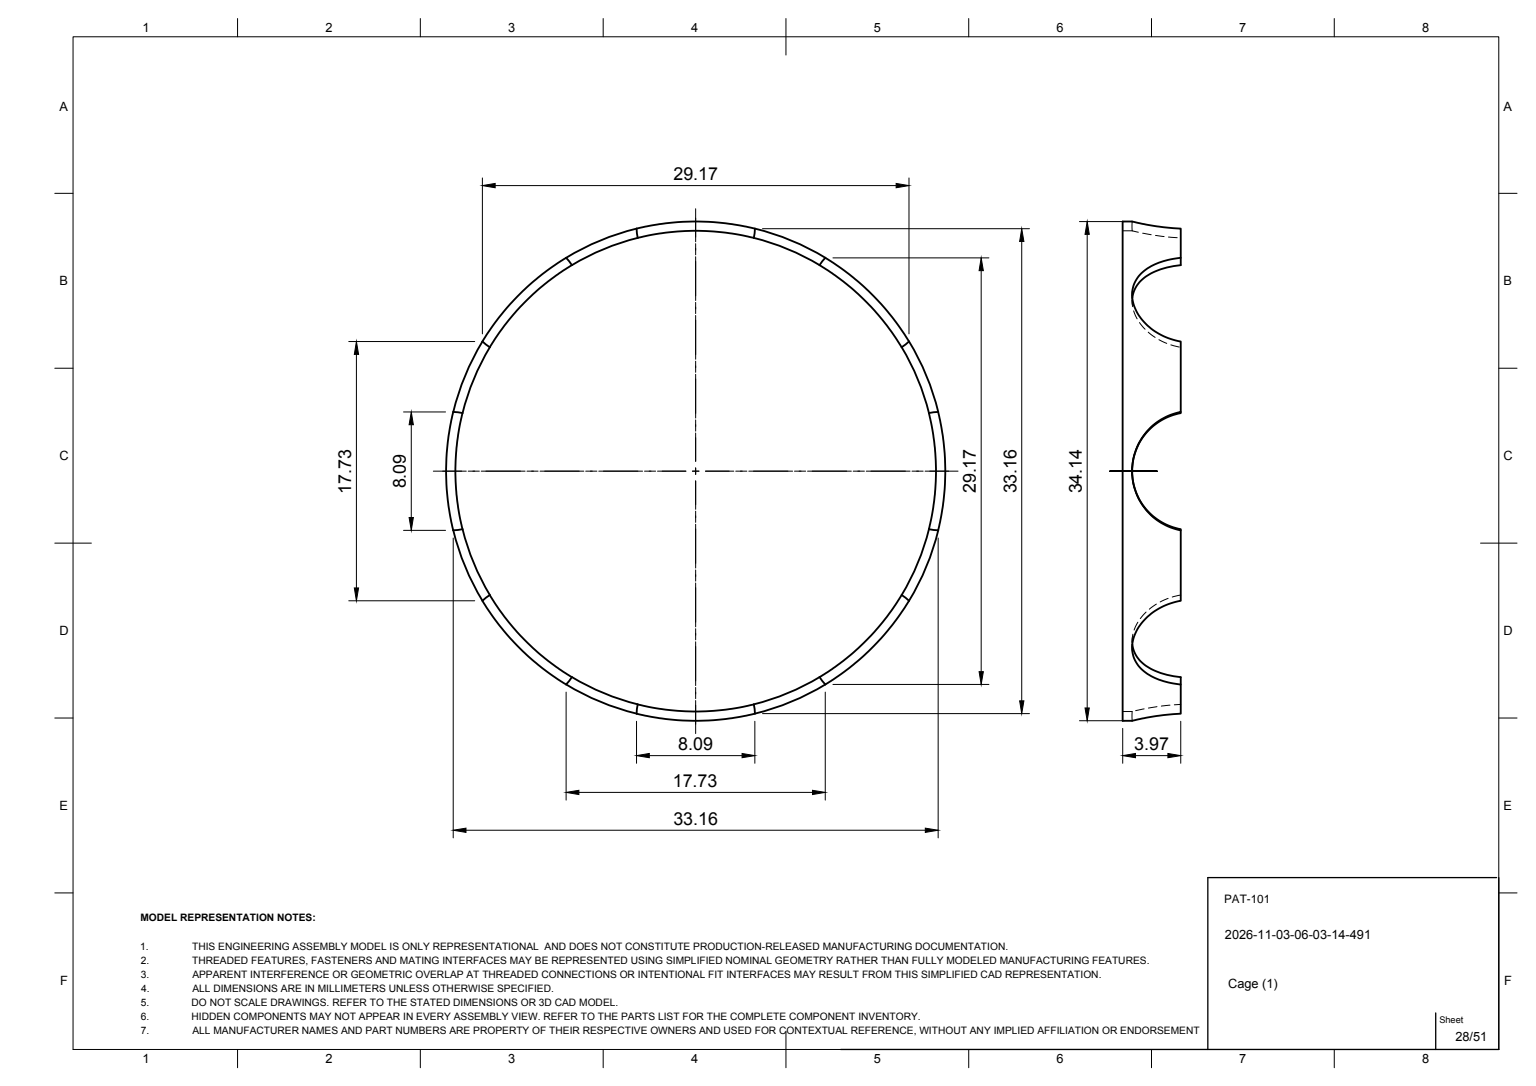
ISO-10303-21;
HEADER;
/* Generated by software containing ST-Developer
 * from STEP Tools, Inc. (www.steptools.com) 
 */

FILE_DESCRIPTION(
/* description */ ('Spur gear reduction stage 2-1 on bearing plates'),
/* implementation_level */ '2;1');

FILE_NAME(
/* name */ 'Cage (1).step',
/* time_stamp */ '2026-10-28T03:22:07-07:00',
/* author */ (''),
/* organization */ (''),
/* preprocessor_version */ 'ST-DEVELOPER v20.2',
/* originating_system */ 'Autodesk Translation Framework v15.17.0.0',
/* authorisation */ '');

FILE_SCHEMA (('AUTOMOTIVE_DESIGN { 1 0 10303 214 3 1 1 }'));
ENDSEC;

DATA;
#10=MECHANICAL_DESIGN_GEOMETRIC_PRESENTATION_REPRESENTATION('',(#982),#53909);
#681=B_SPLINE_CURVE_WITH_KNOTS('',3,(#17332,#17333,#17334,#17335,#17336,
#17337,#17338,#17339,#17340,#17341,#17342,#17343,#17344,#17345,#17346,#17347,
#17348,#17349,#17350,#17351,#17352,#17353),.UNSPECIFIED.,.F.,.F.,(4,2,2,
2,2,2,2,2,2,2,4),(0.0789094028588958,0.210573405340968,0.315860108011452,
0.421146810681936,0.522142632548711,0.623138454415485,0.72413427628226,
0.825130098149035,0.930416800819519,1.03570350349,1.16736750597208),
 .UNSPECIFIED.);
#682=B_SPLINE_CURVE_WITH_KNOTS('',3,(#17357,#17358,#17359,#17360,#17361,
#17362,#17363,#17364,#17365,#17366,#17367,#17368,#17369,#17370,#17371,#17372,
#17373,#17374,#17375,#17376,#17377,#17378),.UNSPECIFIED.,.F.,.F.,(4,2,2,
2,2,2,2,2,2,2,4),(0.0774793363974613,0.142088896491891,0.284177792983782,
0.411119756996526,0.514392970548519,0.617666184100513,0.720939397652506,
0.8242126112045,0.951154575217244,1.09324347170913,1.15785303180356),
 .UNSPECIFIED.);
#683=B_SPLINE_CURVE_WITH_KNOTS('',3,(#17384,#17385,#17386,#17387,#17388,
#17389,#17390,#17391,#17392,#17393,#17394,#17395,#17396,#17397,#17398,#17399,
#17400,#17401,#17402,#17403,#17404,#17405),.UNSPECIFIED.,.F.,.F.,(4,2,2,
2,2,2,2,2,2,2,4),(0.0774793363974613,0.142088896491891,0.284177792983782,
0.411119756996525,0.514392970548519,0.617666184100513,0.720939397652506,
0.8242126112045,0.951154575217243,1.09324347170913,1.15785303180356),
 .UNSPECIFIED.);
#684=B_SPLINE_CURVE_WITH_KNOTS('',3,(#17409,#17410,#17411,#17412,#17413,
#17414,#17415,#17416,#17417,#17418,#17419,#17420,#17421,#17422,#17423,#17424,
#17425,#17426,#17427,#17428,#17429,#17430),.UNSPECIFIED.,.F.,.F.,(4,2,2,
2,2,2,2,2,2,2,4),(0.0774793363974614,0.142088896491891,0.284177792983781,
0.411119756996525,0.514392970548519,0.617666184100512,0.720939397652506,
0.824212611204499,0.951154575217243,1.09324347170913,1.15785303180356),
 .UNSPECIFIED.);
#685=B_SPLINE_CURVE_WITH_KNOTS('',3,(#17434,#17435,#17436,#17437,#17438,
#17439,#17440,#17441,#17442,#17443,#17444,#17445),.UNSPECIFIED.,.F.,.F.,
(4,2,2,2,2,4),(0.0774793363974613,0.142088896491891,0.284177792983781,0.411119756996525,
0.514392970548519,0.617666184100512),.UNSPECIFIED.);
#686=B_SPLINE_CURVE_WITH_KNOTS('',3,(#17450,#17451,#17452,#17453,#17454,
#17455,#17456,#17457,#17458,#17459,#17460,#17461),.UNSPECIFIED.,.F.,.F.,
(4,2,2,2,2,4),(0.617666184100512,0.720939397652506,0.824212611204499,0.951154575217243,
1.09324347170913,1.15785303180356),.UNSPECIFIED.);
#687=B_SPLINE_CURVE_WITH_KNOTS('',3,(#17465,#17466,#17467,#17468,#17469,
#17470,#17471,#17472,#17473,#17474,#17475,#17476,#17477,#17478,#17479,#17480,
#17481,#17482,#17483,#17484,#17485,#17486),.UNSPECIFIED.,.F.,.F.,(4,2,2,
2,2,2,2,2,2,2,4),(0.0774793363974613,0.142088896491891,0.284177792983782,
0.411119756996526,0.514392970548519,0.617666184100513,0.720939397652507,
0.8242126112045,0.951154575217245,1.09324347170914,1.15785303180356),
 .UNSPECIFIED.);
#688=B_SPLINE_CURVE_WITH_KNOTS('',3,(#17490,#17491,#17492,#17493,#17494,
#17495,#17496,#17497,#17498,#17499,#17500,#17501,#17502,#17503,#17504,#17505,
#17506,#17507,#17508,#17509,#17510,#17511),.UNSPECIFIED.,.F.,.F.,(4,2,2,
2,2,2,2,2,2,2,4),(0.0774793363974613,0.142088896491891,0.284177792983782,
0.411119756996526,0.514392970548519,0.617666184100513,0.720939397652506,
0.824212611204499,0.951154575217243,1.09324347170913,1.15785303180356),
 .UNSPECIFIED.);
#689=B_SPLINE_CURVE_WITH_KNOTS('',3,(#17515,#17516,#17517,#17518,#17519,
#17520,#17521,#17522,#17523,#17524,#17525,#17526,#17527,#17528,#17529,#17530,
#17531,#17532,#17533,#17534,#17535,#17536),.UNSPECIFIED.,.F.,.F.,(4,2,2,
2,2,2,2,2,2,2,4),(0.0774793363974613,0.142088896491891,0.284177792983782,
0.411119756996526,0.514392970548519,0.617666184100513,0.720939397652506,
0.8242126112045,0.951154575217244,1.09324347170913,1.15785303180356),
 .UNSPECIFIED.);
#690=B_SPLINE_CURVE_WITH_KNOTS('',3,(#17540,#17541,#17542,#17543,#17544,
#17545,#17546,#17547,#17548,#17549,#17550,#17551,#17552,#17553,#17554,#17555,
#17556,#17557,#17558,#17559,#17560,#17561),.UNSPECIFIED.,.F.,.F.,(4,2,2,
2,2,2,2,2,2,2,4),(0.0774793363974613,0.142088896491891,0.284177792983782,
0.411119756996526,0.514392970548519,0.617666184100513,0.720939397652506,
0.8242126112045,0.951154575217243,1.09324347170913,1.15785303180356),
 .UNSPECIFIED.);
#691=B_SPLINE_CURVE_WITH_KNOTS('',3,(#17569,#17570,#17571,#17572,#17573,
#17574,#17575,#17576,#17577,#17578,#17579,#17580,#17581,#17582,#17583,#17584,
#17585,#17586,#17587,#17588,#17589,#17590),.UNSPECIFIED.,.F.,.F.,(4,2,2,
2,2,2,2,2,2,2,4),(0.0789094028588958,0.210573405340968,0.315860108011452,
0.421146810681936,0.522142632548711,0.623138454415485,0.72413427628226,
0.825130098149035,0.930416800819519,1.03570350349,1.16736750597208),
 .UNSPECIFIED.);
#692=B_SPLINE_CURVE_WITH_KNOTS('',3,(#17598,#17599,#17600,#17601,#17602,
#17603,#17604,#17605,#17606,#17607,#17608,#17609,#17610,#17611,#17612,#17613,
#17614,#17615,#17616,#17617,#17618,#17619),.UNSPECIFIED.,.F.,.F.,(4,2,2,
2,2,2,2,2,2,2,4),(0.0789094028588958,0.210573405340969,0.315860108011453,
0.421146810681937,0.522142632548712,0.623138454415486,0.724134276282261,
0.825130098149035,0.930416800819519,1.03570350349,1.16736750597208),
 .UNSPECIFIED.);
#693=B_SPLINE_CURVE_WITH_KNOTS('',3,(#17628,#17629,#17630,#17631,#17632,
#17633,#17634,#17635,#17636,#17637,#17638,#17639),.UNSPECIFIED.,.F.,.F.,
(4,2,2,2,2,4),(0.0789094028588958,0.210573405340968,0.315860108011452,0.421146810681937,
0.522142632548711,0.623138454415486),.UNSPECIFIED.);
#694=B_SPLINE_CURVE_WITH_KNOTS('',3,(#17641,#17642,#17643,#17644,#17645,
#17646,#17647,#17648,#17649,#17650,#17651,#17652),.UNSPECIFIED.,.F.,.F.,
(4,2,2,2,2,4),(0.623138454415486,0.72413427628226,0.825130098149035,0.930416800819519,
1.03570350349,1.16736750597208),.UNSPECIFIED.);
#695=B_SPLINE_CURVE_WITH_KNOTS('',3,(#17659,#17660,#17661,#17662,#17663,
#17664,#17665,#17666,#17667,#17668,#17669,#17670,#17671,#17672,#17673,#17674,
#17675,#17676,#17677,#17678,#17679,#17680),.UNSPECIFIED.,.F.,.F.,(4,2,2,
2,2,2,2,2,2,2,4),(0.0789094028588958,0.210573405340968,0.315860108011452,
0.421146810681936,0.522142632548711,0.623138454415486,0.72413427628226,
0.825130098149035,0.930416800819519,1.03570350349,1.16736750597208),
 .UNSPECIFIED.);
#696=B_SPLINE_CURVE_WITH_KNOTS('',3,(#17688,#17689,#17690,#17691,#17692,
#17693,#17694,#17695,#17696,#17697,#17698,#17699,#17700,#17701,#17702,#17703,
#17704,#17705,#17706,#17707,#17708,#17709),.UNSPECIFIED.,.F.,.F.,(4,2,2,
2,2,2,2,2,2,2,4),(0.0789094028588957,0.210573405340968,0.315860108011452,
0.421146810681936,0.522142632548711,0.623138454415485,0.72413427628226,
0.825130098149035,0.930416800819519,1.03570350349,1.16736750597207),
 .UNSPECIFIED.);
#697=B_SPLINE_CURVE_WITH_KNOTS('',3,(#17717,#17718,#17719,#17720,#17721,
#17722,#17723,#17724,#17725,#17726,#17727,#17728,#17729,#17730,#17731,#17732,
#17733,#17734,#17735,#17736,#17737,#17738),.UNSPECIFIED.,.F.,.F.,(4,2,2,
2,2,2,2,2,2,2,4),(0.0789094028588958,0.210573405340968,0.315860108011452,
0.421146810681936,0.522142632548711,0.623138454415486,0.72413427628226,
0.825130098149035,0.930416800819519,1.03570350349,1.16736750597208),
 .UNSPECIFIED.);
#698=B_SPLINE_CURVE_WITH_KNOTS('',3,(#17747,#17748,#17749,#17750,#17751,
#17752,#17753,#17754,#17755,#17756,#17757,#17758,#17759,#17760,#17761,#17762,
#17763,#17764,#17765,#17766,#17767,#17768),.UNSPECIFIED.,.F.,.F.,(4,2,2,
2,2,2,2,2,2,2,4),(0.0789094028588958,0.210573405340968,0.315860108011452,
0.421146810681936,0.522142632548711,0.623138454415485,0.72413427628226,
0.825130098149035,0.930416800819519,1.03570350349,1.16736750597208),
 .UNSPECIFIED.);
#817=SPHERICAL_SURFACE('',#12340,0.412776);
#818=SPHERICAL_SURFACE('',#12356,0.412776);
#819=SPHERICAL_SURFACE('',#12361,0.412776);
#820=SPHERICAL_SURFACE('',#12366,0.412776);
#821=SPHERICAL_SURFACE('',#12371,0.412776);
#822=SPHERICAL_SURFACE('',#12376,0.412776);
#823=SPHERICAL_SURFACE('',#12381,0.412776);
#824=SPHERICAL_SURFACE('',#12389,0.412776);
#882=SHAPE_REPRESENTATION_RELATIONSHIP('SRR','None',#54111,#925);
#925=ADVANCED_BREP_SHAPE_REPRESENTATION('',(#1038),#53885);
#982=STYLED_ITEM('',(#54397),#1038);
#1038=MANIFOLD_SOLID_BREP('Continuous crown cage',#11308);
#1191=FACE_BOUND('',#2536,.T.);
#1334=PLANE('',#12353);
#1335=PLANE('',#12358);
#1336=PLANE('',#12363);
#1337=PLANE('',#12368);
#1338=PLANE('',#12373);
#1339=PLANE('',#12378);
#1340=PLANE('',#12387);
#1341=PLANE('',#12391);
#1342=PLANE('',#12392);
#1739=FACE_OUTER_BOUND('',#2518,.T.);
#1740=FACE_OUTER_BOUND('',#2519,.T.);
#1741=FACE_OUTER_BOUND('',#2520,.T.);
#1742=FACE_OUTER_BOUND('',#2521,.T.);
#1743=FACE_OUTER_BOUND('',#2522,.T.);
#1744=FACE_OUTER_BOUND('',#2523,.T.);
#1745=FACE_OUTER_BOUND('',#2524,.T.);
#1746=FACE_OUTER_BOUND('',#2525,.T.);
#1747=FACE_OUTER_BOUND('',#2526,.T.);
#1748=FACE_OUTER_BOUND('',#2527,.T.);
#1749=FACE_OUTER_BOUND('',#2528,.T.);
#1750=FACE_OUTER_BOUND('',#2529,.T.);
#1751=FACE_OUTER_BOUND('',#2530,.T.);
#1752=FACE_OUTER_BOUND('',#2531,.T.);
#1753=FACE_OUTER_BOUND('',#2532,.T.);
#1754=FACE_OUTER_BOUND('',#2533,.T.);
#1755=FACE_OUTER_BOUND('',#2534,.T.);
#1756=FACE_OUTER_BOUND('',#2535,.T.);
#1757=FACE_OUTER_BOUND('',#2537,.T.);
#2518=EDGE_LOOP('',(#8286,#8287,#8288,#8289));
#2519=EDGE_LOOP('',(#8290,#8291,#8292,#8293,#8294,#8295,#8296,#8297,#8298,
#8299,#8300,#8301,#8302,#8303,#8304,#8305,#8306,#8307,#8308,#8309));
#2520=EDGE_LOOP('',(#8310,#8311,#8312,#8313));
#2521=EDGE_LOOP('',(#8314,#8315,#8316,#8317));
#2522=EDGE_LOOP('',(#8318,#8319,#8320,#8321));
#2523=EDGE_LOOP('',(#8322,#8323,#8324,#8325));
#2524=EDGE_LOOP('',(#8326,#8327,#8328,#8329));
#2525=EDGE_LOOP('',(#8330,#8331,#8332,#8333,#8334,#8335));
#2526=EDGE_LOOP('',(#8336,#8337,#8338,#8339));
#2527=EDGE_LOOP('',(#8340,#8341,#8342,#8343));
#2528=EDGE_LOOP('',(#8344,#8345,#8346,#8347));
#2529=EDGE_LOOP('',(#8348,#8349,#8350,#8351));
#2530=EDGE_LOOP('',(#8352,#8353,#8354,#8355));
#2531=EDGE_LOOP('',(#8356,#8357,#8358,#8359));
#2532=EDGE_LOOP('',(#8360,#8361,#8362,#8363,#8364,#8365,#8366,#8367,#8368,
#8369,#8370,#8371,#8372,#8373,#8374,#8375,#8376,#8377,#8378,#8379));
#2533=EDGE_LOOP('',(#8380,#8381,#8382,#8383));
#2534=EDGE_LOOP('',(#8384,#8385,#8386,#8387));
#2535=EDGE_LOOP('',(#8388));
#2536=EDGE_LOOP('',(#8389));
#2537=EDGE_LOOP('',(#8390,#8391,#8392,#8393));
#3163=LINE('',#17447,#3804);
#3164=LINE('',#17743,#3805);
#3804=VECTOR('',#14250,1.706752);
#3805=VECTOR('',#14327,1.643248);
#4526=CIRCLE('',#12341,0.405071403305639);
#4527=CIRCLE('',#12342,0.405071403305639);
#4528=CIRCLE('',#12344,1.706752);
#4529=CIRCLE('',#12345,1.706752);
#4530=CIRCLE('',#12346,1.706752);
#4531=CIRCLE('',#12347,1.706752);
#4532=CIRCLE('',#12348,1.706752);
#4533=CIRCLE('',#12349,1.706752);
#4534=CIRCLE('',#12350,1.706752);
#4535=CIRCLE('',#12351,1.706752);
#4536=CIRCLE('',#12352,1.706752);
#4537=CIRCLE('',#12354,1.643248);
#4538=CIRCLE('',#12355,0.405071403305639);
#4539=CIRCLE('',#12357,0.405071403305639);
#4540=CIRCLE('',#12359,1.643248);
#4541=CIRCLE('',#12360,0.405071403305639);
#4542=CIRCLE('',#12362,0.405071403305639);
#4543=CIRCLE('',#12364,1.643248);
#4544=CIRCLE('',#12365,0.405071403305639);
#4545=CIRCLE('',#12367,0.405071403305639);
#4546=CIRCLE('',#12369,1.643248);
#4547=CIRCLE('',#12370,0.405071403305639);
#4548=CIRCLE('',#12372,0.405071403305639);
#4549=CIRCLE('',#12374,1.643248);
#4550=CIRCLE('',#12375,0.405071403305639);
#4551=CIRCLE('',#12377,0.405071403305639);
#4552=CIRCLE('',#12379,1.643248);
#4553=CIRCLE('',#12380,0.405071403305639);
#4554=CIRCLE('',#12382,0.405071403305639);
#4555=CIRCLE('',#12384,1.643248);
#4556=CIRCLE('',#12385,1.643248);
#4557=CIRCLE('',#12386,1.643248);
#4558=CIRCLE('',#12388,0.405071403305639);
#4559=CIRCLE('',#12390,0.405071403305639);
#5110=VERTEX_POINT('',#17330);
#5111=VERTEX_POINT('',#17331);
#5112=VERTEX_POINT('',#17354);
#5113=VERTEX_POINT('',#17356);
#5114=VERTEX_POINT('',#17381);
#5115=VERTEX_POINT('',#17383);
#5116=VERTEX_POINT('',#17406);
#5117=VERTEX_POINT('',#17408);
#5118=VERTEX_POINT('',#17431);
#5119=VERTEX_POINT('',#17433);
#5120=VERTEX_POINT('',#17446);
#5121=VERTEX_POINT('',#17449);
#5122=VERTEX_POINT('',#17462);
#5123=VERTEX_POINT('',#17464);
#5124=VERTEX_POINT('',#17487);
#5125=VERTEX_POINT('',#17489);
#5126=VERTEX_POINT('',#17512);
#5127=VERTEX_POINT('',#17514);
#5128=VERTEX_POINT('',#17537);
#5129=VERTEX_POINT('',#17539);
#5130=VERTEX_POINT('',#17564);
#5131=VERTEX_POINT('',#17568);
#5132=VERTEX_POINT('',#17593);
#5133=VERTEX_POINT('',#17597);
#5134=VERTEX_POINT('',#17622);
#5135=VERTEX_POINT('',#17626);
#5136=VERTEX_POINT('',#17627);
#5137=VERTEX_POINT('',#17654);
#5138=VERTEX_POINT('',#17658);
#5139=VERTEX_POINT('',#17683);
#5140=VERTEX_POINT('',#17687);
#5141=VERTEX_POINT('',#17712);
#5142=VERTEX_POINT('',#17716);
#5143=VERTEX_POINT('',#17741);
#5144=VERTEX_POINT('',#17744);
#5145=VERTEX_POINT('',#17746);
#6285=EDGE_CURVE('',#5110,#5111,#681,.T.);
#6286=EDGE_CURVE('',#5112,#5110,#4526,.T.);
#6287=EDGE_CURVE('',#5113,#5112,#682,.T.);
#6288=EDGE_CURVE('',#5111,#5113,#4527,.T.);
#6289=EDGE_CURVE('',#5114,#5112,#4528,.T.);
#6290=EDGE_CURVE('',#5114,#5115,#683,.T.);
#6291=EDGE_CURVE('',#5116,#5115,#4529,.T.);
#6292=EDGE_CURVE('',#5116,#5117,#684,.T.);
#6293=EDGE_CURVE('',#5118,#5117,#4530,.T.);
#6294=EDGE_CURVE('',#5118,#5119,#685,.T.);
#6295=EDGE_CURVE('',#5119,#5120,#3163,.T.);
#6296=EDGE_CURVE('',#5120,#5120,#4531,.T.);
#6297=EDGE_CURVE('',#5119,#5121,#686,.T.);
#6298=EDGE_CURVE('',#5122,#5121,#4532,.T.);
#6299=EDGE_CURVE('',#5122,#5123,#687,.T.);
#6300=EDGE_CURVE('',#5124,#5123,#4533,.T.);
#6301=EDGE_CURVE('',#5124,#5125,#688,.T.);
#6302=EDGE_CURVE('',#5126,#5125,#4534,.T.);
#6303=EDGE_CURVE('',#5126,#5127,#689,.T.);
#6304=EDGE_CURVE('',#5128,#5127,#4535,.T.);
#6305=EDGE_CURVE('',#5128,#5129,#690,.T.);
#6306=EDGE_CURVE('',#5113,#5129,#4536,.T.);
#6307=EDGE_CURVE('',#5110,#5130,#4537,.T.);
#6308=EDGE_CURVE('',#5130,#5114,#4538,.T.);
#6309=EDGE_CURVE('',#5131,#5130,#691,.T.);
#6310=EDGE_CURVE('',#5115,#5131,#4539,.T.);
#6311=EDGE_CURVE('',#5131,#5132,#4540,.T.);
#6312=EDGE_CURVE('',#5132,#5116,#4541,.T.);
#6313=EDGE_CURVE('',#5133,#5132,#692,.T.);
#6314=EDGE_CURVE('',#5117,#5133,#4542,.T.);
#6315=EDGE_CURVE('',#5133,#5134,#4543,.T.);
#6316=EDGE_CURVE('',#5134,#5118,#4544,.T.);
#6317=EDGE_CURVE('',#5135,#5136,#693,.T.);
#6318=EDGE_CURVE('',#5121,#5135,#4545,.T.);
#6319=EDGE_CURVE('',#5136,#5134,#694,.T.);
#6320=EDGE_CURVE('',#5135,#5137,#4546,.T.);
#6321=EDGE_CURVE('',#5137,#5122,#4547,.T.);
#6322=EDGE_CURVE('',#5138,#5137,#695,.T.);
#6323=EDGE_CURVE('',#5123,#5138,#4548,.T.);
#6324=EDGE_CURVE('',#5138,#5139,#4549,.T.);
#6325=EDGE_CURVE('',#5139,#5124,#4550,.T.);
#6326=EDGE_CURVE('',#5140,#5139,#696,.T.);
#6327=EDGE_CURVE('',#5125,#5140,#4551,.T.);
#6328=EDGE_CURVE('',#5140,#5141,#4552,.T.);
#6329=EDGE_CURVE('',#5141,#5126,#4553,.T.);
#6330=EDGE_CURVE('',#5142,#5141,#697,.T.);
#6331=EDGE_CURVE('',#5127,#5142,#4554,.T.);
#6332=EDGE_CURVE('',#5143,#5143,#4555,.T.);
#6333=EDGE_CURVE('',#5143,#5136,#3164,.T.);
#6334=EDGE_CURVE('',#5144,#5111,#4556,.T.);
#6335=EDGE_CURVE('',#5144,#5145,#698,.T.);
#6336=EDGE_CURVE('',#5142,#5145,#4557,.T.);
#6337=EDGE_CURVE('',#5129,#5144,#4558,.T.);
#6338=EDGE_CURVE('',#5145,#5128,#4559,.T.);
#8286=ORIENTED_EDGE('',*,*,#6285,.F.);
#8287=ORIENTED_EDGE('',*,*,#6286,.F.);
#8288=ORIENTED_EDGE('',*,*,#6287,.F.);
#8289=ORIENTED_EDGE('',*,*,#6288,.F.);
#8290=ORIENTED_EDGE('',*,*,#6287,.T.);
#8291=ORIENTED_EDGE('',*,*,#6289,.F.);
#8292=ORIENTED_EDGE('',*,*,#6290,.T.);
#8293=ORIENTED_EDGE('',*,*,#6291,.F.);
#8294=ORIENTED_EDGE('',*,*,#6292,.T.);
#8295=ORIENTED_EDGE('',*,*,#6293,.F.);
#8296=ORIENTED_EDGE('',*,*,#6294,.T.);
#8297=ORIENTED_EDGE('',*,*,#6295,.T.);
#8298=ORIENTED_EDGE('',*,*,#6296,.F.);
#8299=ORIENTED_EDGE('',*,*,#6295,.F.);
#8300=ORIENTED_EDGE('',*,*,#6297,.T.);
#8301=ORIENTED_EDGE('',*,*,#6298,.F.);
#8302=ORIENTED_EDGE('',*,*,#6299,.T.);
#8303=ORIENTED_EDGE('',*,*,#6300,.F.);
#8304=ORIENTED_EDGE('',*,*,#6301,.T.);
#8305=ORIENTED_EDGE('',*,*,#6302,.F.);
#8306=ORIENTED_EDGE('',*,*,#6303,.T.);
#8307=ORIENTED_EDGE('',*,*,#6304,.F.);
#8308=ORIENTED_EDGE('',*,*,#6305,.T.);
#8309=ORIENTED_EDGE('',*,*,#6306,.F.);
#8310=ORIENTED_EDGE('',*,*,#6286,.T.);
#8311=ORIENTED_EDGE('',*,*,#6307,.T.);
#8312=ORIENTED_EDGE('',*,*,#6308,.T.);
#8313=ORIENTED_EDGE('',*,*,#6289,.T.);
#8314=ORIENTED_EDGE('',*,*,#6309,.F.);
#8315=ORIENTED_EDGE('',*,*,#6310,.F.);
#8316=ORIENTED_EDGE('',*,*,#6290,.F.);
#8317=ORIENTED_EDGE('',*,*,#6308,.F.);
#8318=ORIENTED_EDGE('',*,*,#6310,.T.);
#8319=ORIENTED_EDGE('',*,*,#6311,.T.);
#8320=ORIENTED_EDGE('',*,*,#6312,.T.);
#8321=ORIENTED_EDGE('',*,*,#6291,.T.);
#8322=ORIENTED_EDGE('',*,*,#6313,.F.);
#8323=ORIENTED_EDGE('',*,*,#6314,.F.);
#8324=ORIENTED_EDGE('',*,*,#6292,.F.);
#8325=ORIENTED_EDGE('',*,*,#6312,.F.);
#8326=ORIENTED_EDGE('',*,*,#6314,.T.);
#8327=ORIENTED_EDGE('',*,*,#6315,.T.);
#8328=ORIENTED_EDGE('',*,*,#6316,.T.);
#8329=ORIENTED_EDGE('',*,*,#6293,.T.);
#8330=ORIENTED_EDGE('',*,*,#6317,.F.);
#8331=ORIENTED_EDGE('',*,*,#6318,.F.);
#8332=ORIENTED_EDGE('',*,*,#6297,.F.);
#8333=ORIENTED_EDGE('',*,*,#6294,.F.);
#8334=ORIENTED_EDGE('',*,*,#6316,.F.);
#8335=ORIENTED_EDGE('',*,*,#6319,.F.);
#8336=ORIENTED_EDGE('',*,*,#6318,.T.);
#8337=ORIENTED_EDGE('',*,*,#6320,.T.);
#8338=ORIENTED_EDGE('',*,*,#6321,.T.);
#8339=ORIENTED_EDGE('',*,*,#6298,.T.);
#8340=ORIENTED_EDGE('',*,*,#6322,.F.);
#8341=ORIENTED_EDGE('',*,*,#6323,.F.);
#8342=ORIENTED_EDGE('',*,*,#6299,.F.);
#8343=ORIENTED_EDGE('',*,*,#6321,.F.);
#8344=ORIENTED_EDGE('',*,*,#6323,.T.);
#8345=ORIENTED_EDGE('',*,*,#6324,.T.);
#8346=ORIENTED_EDGE('',*,*,#6325,.T.);
#8347=ORIENTED_EDGE('',*,*,#6300,.T.);
#8348=ORIENTED_EDGE('',*,*,#6326,.F.);
#8349=ORIENTED_EDGE('',*,*,#6327,.F.);
#8350=ORIENTED_EDGE('',*,*,#6301,.F.);
#8351=ORIENTED_EDGE('',*,*,#6325,.F.);
#8352=ORIENTED_EDGE('',*,*,#6327,.T.);
#8353=ORIENTED_EDGE('',*,*,#6328,.T.);
#8354=ORIENTED_EDGE('',*,*,#6329,.T.);
#8355=ORIENTED_EDGE('',*,*,#6302,.T.);
#8356=ORIENTED_EDGE('',*,*,#6303,.F.);
#8357=ORIENTED_EDGE('',*,*,#6329,.F.);
#8358=ORIENTED_EDGE('',*,*,#6330,.F.);
#8359=ORIENTED_EDGE('',*,*,#6331,.F.);
#8360=ORIENTED_EDGE('',*,*,#6332,.F.);
#8361=ORIENTED_EDGE('',*,*,#6333,.T.);
#8362=ORIENTED_EDGE('',*,*,#6319,.T.);
#8363=ORIENTED_EDGE('',*,*,#6315,.F.);
#8364=ORIENTED_EDGE('',*,*,#6313,.T.);
#8365=ORIENTED_EDGE('',*,*,#6311,.F.);
#8366=ORIENTED_EDGE('',*,*,#6309,.T.);
#8367=ORIENTED_EDGE('',*,*,#6307,.F.);
#8368=ORIENTED_EDGE('',*,*,#6285,.T.);
#8369=ORIENTED_EDGE('',*,*,#6334,.F.);
#8370=ORIENTED_EDGE('',*,*,#6335,.T.);
#8371=ORIENTED_EDGE('',*,*,#6336,.F.);
#8372=ORIENTED_EDGE('',*,*,#6330,.T.);
#8373=ORIENTED_EDGE('',*,*,#6328,.F.);
#8374=ORIENTED_EDGE('',*,*,#6326,.T.);
#8375=ORIENTED_EDGE('',*,*,#6324,.F.);
#8376=ORIENTED_EDGE('',*,*,#6322,.T.);
#8377=ORIENTED_EDGE('',*,*,#6320,.F.);
#8378=ORIENTED_EDGE('',*,*,#6317,.T.);
#8379=ORIENTED_EDGE('',*,*,#6333,.F.);
#8380=ORIENTED_EDGE('',*,*,#6288,.T.);
#8381=ORIENTED_EDGE('',*,*,#6306,.T.);
#8382=ORIENTED_EDGE('',*,*,#6337,.T.);
#8383=ORIENTED_EDGE('',*,*,#6334,.T.);
#8384=ORIENTED_EDGE('',*,*,#6305,.F.);
#8385=ORIENTED_EDGE('',*,*,#6338,.F.);
#8386=ORIENTED_EDGE('',*,*,#6335,.F.);
#8387=ORIENTED_EDGE('',*,*,#6337,.F.);
#8388=ORIENTED_EDGE('',*,*,#6296,.T.);
#8389=ORIENTED_EDGE('',*,*,#6332,.T.);
#8390=ORIENTED_EDGE('',*,*,#6331,.T.);
#8391=ORIENTED_EDGE('',*,*,#6336,.T.);
#8392=ORIENTED_EDGE('',*,*,#6338,.T.);
#8393=ORIENTED_EDGE('',*,*,#6304,.T.);
#10518=CYLINDRICAL_SURFACE('',#12343,1.706752);
#10519=CYLINDRICAL_SURFACE('',#12383,1.643248);
#10859=ADVANCED_FACE('',(#1739),#817,.F.);
#10860=ADVANCED_FACE('',(#1740),#10518,.T.);
#10861=ADVANCED_FACE('',(#1741),#1334,.T.);
#10862=ADVANCED_FACE('',(#1742),#818,.F.);
#10863=ADVANCED_FACE('',(#1743),#1335,.T.);
#10864=ADVANCED_FACE('',(#1744),#819,.F.);
#10865=ADVANCED_FACE('',(#1745),#1336,.T.);
#10866=ADVANCED_FACE('',(#1746),#820,.F.);
#10867=ADVANCED_FACE('',(#1747),#1337,.T.);
#10868=ADVANCED_FACE('',(#1748),#821,.F.);
#10869=ADVANCED_FACE('',(#1749),#1338,.T.);
#10870=ADVANCED_FACE('',(#1750),#822,.F.);
#10871=ADVANCED_FACE('',(#1751),#1339,.T.);
#10872=ADVANCED_FACE('',(#1752),#823,.F.);
#10873=ADVANCED_FACE('',(#1753),#10519,.F.);
#10874=ADVANCED_FACE('',(#1754),#1340,.T.);
#10875=ADVANCED_FACE('',(#1755),#824,.F.);
#10876=ADVANCED_FACE('',(#1756,#1191),#1341,.T.);
#10877=ADVANCED_FACE('',(#1757),#1342,.T.);
#11308=CLOSED_SHELL('',(#10859,#10860,#10861,#10862,#10863,#10864,#10865,
#10866,#10867,#10868,#10869,#10870,#10871,#10872,#10873,#10874,#10875,#10876,
#10877));
#12339=AXIS2_PLACEMENT_3D('',#17328,#14234,#14235);
#12340=AXIS2_PLACEMENT_3D('',#17329,#14236,#14237);
#12341=AXIS2_PLACEMENT_3D('',#17355,#14238,#14239);
#12342=AXIS2_PLACEMENT_3D('',#17379,#14240,#14241);
#12343=AXIS2_PLACEMENT_3D('',#17380,#14242,#14243);
#12344=AXIS2_PLACEMENT_3D('',#17382,#14244,#14245);
#12345=AXIS2_PLACEMENT_3D('',#17407,#14246,#14247);
#12346=AXIS2_PLACEMENT_3D('',#17432,#14248,#14249);
#12347=AXIS2_PLACEMENT_3D('',#17448,#14251,#14252);
#12348=AXIS2_PLACEMENT_3D('',#17463,#14253,#14254);
#12349=AXIS2_PLACEMENT_3D('',#17488,#14255,#14256);
#12350=AXIS2_PLACEMENT_3D('',#17513,#14257,#14258);
#12351=AXIS2_PLACEMENT_3D('',#17538,#14259,#14260);
#12352=AXIS2_PLACEMENT_3D('',#17562,#14261,#14262);
#12353=AXIS2_PLACEMENT_3D('',#17563,#14263,#14264);
#12354=AXIS2_PLACEMENT_3D('',#17565,#14265,#14266);
#12355=AXIS2_PLACEMENT_3D('',#17566,#14267,#14268);
#12356=AXIS2_PLACEMENT_3D('',#17567,#14269,#14270);
#12357=AXIS2_PLACEMENT_3D('',#17591,#14271,#14272);
#12358=AXIS2_PLACEMENT_3D('',#17592,#14273,#14274);
#12359=AXIS2_PLACEMENT_3D('',#17594,#14275,#14276);
#12360=AXIS2_PLACEMENT_3D('',#17595,#14277,#14278);
#12361=AXIS2_PLACEMENT_3D('',#17596,#14279,#14280);
#12362=AXIS2_PLACEMENT_3D('',#17620,#14281,#14282);
#12363=AXIS2_PLACEMENT_3D('',#17621,#14283,#14284);
#12364=AXIS2_PLACEMENT_3D('',#17623,#14285,#14286);
#12365=AXIS2_PLACEMENT_3D('',#17624,#14287,#14288);
#12366=AXIS2_PLACEMENT_3D('',#17625,#14289,#14290);
#12367=AXIS2_PLACEMENT_3D('',#17640,#14291,#14292);
#12368=AXIS2_PLACEMENT_3D('',#17653,#14293,#14294);
#12369=AXIS2_PLACEMENT_3D('',#17655,#14295,#14296);
#12370=AXIS2_PLACEMENT_3D('',#17656,#14297,#14298);
#12371=AXIS2_PLACEMENT_3D('',#17657,#14299,#14300);
#12372=AXIS2_PLACEMENT_3D('',#17681,#14301,#14302);
#12373=AXIS2_PLACEMENT_3D('',#17682,#14303,#14304);
#12374=AXIS2_PLACEMENT_3D('',#17684,#14305,#14306);
#12375=AXIS2_PLACEMENT_3D('',#17685,#14307,#14308);
#12376=AXIS2_PLACEMENT_3D('',#17686,#14309,#14310);
#12377=AXIS2_PLACEMENT_3D('',#17710,#14311,#14312);
#12378=AXIS2_PLACEMENT_3D('',#17711,#14313,#14314);
#12379=AXIS2_PLACEMENT_3D('',#17713,#14315,#14316);
#12380=AXIS2_PLACEMENT_3D('',#17714,#14317,#14318);
#12381=AXIS2_PLACEMENT_3D('',#17715,#14319,#14320);
#12382=AXIS2_PLACEMENT_3D('',#17739,#14321,#14322);
#12383=AXIS2_PLACEMENT_3D('',#17740,#14323,#14324);
#12384=AXIS2_PLACEMENT_3D('',#17742,#14325,#14326);
#12385=AXIS2_PLACEMENT_3D('',#17745,#14328,#14329);
#12386=AXIS2_PLACEMENT_3D('',#17769,#14330,#14331);
#12387=AXIS2_PLACEMENT_3D('',#17770,#14332,#14333);
#12388=AXIS2_PLACEMENT_3D('',#17771,#14334,#14335);
#12389=AXIS2_PLACEMENT_3D('',#17772,#14336,#14337);
#12390=AXIS2_PLACEMENT_3D('',#17773,#14338,#14339);
#12391=AXIS2_PLACEMENT_3D('',#17774,#14340,#14341);
#12392=AXIS2_PLACEMENT_3D('',#17775,#14342,#14343);
#14234=DIRECTION('axis',(0.,0.,1.));
#14235=DIRECTION('refdir',(1.,0.,0.));
#14236=DIRECTION('center_axis',(0.,0.,1.));
#14237=DIRECTION('ref_axis',(1.,0.,0.));
#14238=DIRECTION('center_axis',(0.,-1.,0.));
#14239=DIRECTION('ref_axis',(0.,0.,-1.));
#14240=DIRECTION('center_axis',(0.,-1.,0.));
#14241=DIRECTION('ref_axis',(0.,0.,-1.));
#14242=DIRECTION('center_axis',(0.,1.,0.));
#14243=DIRECTION('ref_axis',(1.,0.,0.));
#14244=DIRECTION('center_axis',(0.,1.,0.));
#14245=DIRECTION('ref_axis',(1.,0.,0.));
#14246=DIRECTION('center_axis',(0.,1.,0.));
#14247=DIRECTION('ref_axis',(1.,0.,0.));
#14248=DIRECTION('center_axis',(0.,1.,0.));
#14249=DIRECTION('ref_axis',(1.,0.,0.));
#14250=DIRECTION('',(0.,-1.,0.));
#14251=DIRECTION('center_axis',(0.,-1.,0.));
#14252=DIRECTION('ref_axis',(1.,0.,0.));
#14253=DIRECTION('center_axis',(0.,1.,0.));
#14254=DIRECTION('ref_axis',(1.,0.,0.));
#14255=DIRECTION('center_axis',(0.,1.,0.));
#14256=DIRECTION('ref_axis',(1.,0.,0.));
#14257=DIRECTION('center_axis',(0.,1.,0.));
#14258=DIRECTION('ref_axis',(1.,0.,0.));
#14259=DIRECTION('center_axis',(0.,1.,0.));
#14260=DIRECTION('ref_axis',(1.,0.,0.));
#14261=DIRECTION('center_axis',(0.,1.,0.));
#14262=DIRECTION('ref_axis',(1.,0.,0.));
#14263=DIRECTION('center_axis',(0.,1.,0.));
#14264=DIRECTION('ref_axis',(1.,0.,0.));
#14265=DIRECTION('center_axis',(0.,-1.,0.));
#14266=DIRECTION('ref_axis',(1.,0.,0.));
#14267=DIRECTION('center_axis',(0.,-1.,0.));
#14268=DIRECTION('ref_axis',(0.,0.,-1.));
#14269=DIRECTION('center_axis',(6.12323399573677E-17,0.,1.));
#14270=DIRECTION('ref_axis',(1.,0.,0.));
#14271=DIRECTION('center_axis',(0.,-1.,0.));
#14272=DIRECTION('ref_axis',(0.,0.,-1.));
#14273=DIRECTION('center_axis',(0.,1.,0.));
#14274=DIRECTION('ref_axis',(1.,0.,0.));
#14275=DIRECTION('center_axis',(0.,-1.,0.));
#14276=DIRECTION('ref_axis',(1.,0.,0.));
#14277=DIRECTION('center_axis',(0.,-1.,0.));
#14278=DIRECTION('ref_axis',(0.,0.,-1.));
#14279=DIRECTION('center_axis',(0.,0.,1.));
#14280=DIRECTION('ref_axis',(1.,0.,0.));
#14281=DIRECTION('center_axis',(0.,-1.,0.));
#14282=DIRECTION('ref_axis',(0.,0.,-1.));
#14283=DIRECTION('center_axis',(0.,1.,0.));
#14284=DIRECTION('ref_axis',(1.,0.,0.));
#14285=DIRECTION('center_axis',(0.,-1.,0.));
#14286=DIRECTION('ref_axis',(1.,0.,0.));
#14287=DIRECTION('center_axis',(0.,-1.,0.));
#14288=DIRECTION('ref_axis',(0.,0.,-1.));
#14289=DIRECTION('center_axis',(0.,0.,1.));
#14290=DIRECTION('ref_axis',(1.,0.,0.));
#14291=DIRECTION('center_axis',(0.,-1.,0.));
#14292=DIRECTION('ref_axis',(0.,0.,-1.));
#14293=DIRECTION('center_axis',(0.,1.,0.));
#14294=DIRECTION('ref_axis',(1.,0.,0.));
#14295=DIRECTION('center_axis',(0.,-1.,0.));
#14296=DIRECTION('ref_axis',(1.,0.,0.));
#14297=DIRECTION('center_axis',(0.,-1.,0.));
#14298=DIRECTION('ref_axis',(0.,0.,-1.));
#14299=DIRECTION('center_axis',(0.,0.,1.));
#14300=DIRECTION('ref_axis',(1.,0.,0.));
#14301=DIRECTION('center_axis',(0.,-1.,0.));
#14302=DIRECTION('ref_axis',(0.,0.,-1.));
#14303=DIRECTION('center_axis',(0.,1.,0.));
#14304=DIRECTION('ref_axis',(1.,0.,0.));
#14305=DIRECTION('center_axis',(0.,-1.,0.));
#14306=DIRECTION('ref_axis',(1.,0.,0.));
#14307=DIRECTION('center_axis',(0.,-1.,0.));
#14308=DIRECTION('ref_axis',(0.,0.,-1.));
#14309=DIRECTION('center_axis',(6.12323399573676E-17,0.,1.));
#14310=DIRECTION('ref_axis',(1.,0.,0.));
#14311=DIRECTION('center_axis',(0.,-1.,0.));
#14312=DIRECTION('ref_axis',(0.,0.,-1.));
#14313=DIRECTION('center_axis',(0.,1.,0.));
#14314=DIRECTION('ref_axis',(1.,0.,0.));
#14315=DIRECTION('center_axis',(0.,-1.,0.));
#14316=DIRECTION('ref_axis',(1.,0.,0.));
#14317=DIRECTION('center_axis',(0.,-1.,0.));
#14318=DIRECTION('ref_axis',(0.,0.,-1.));
#14319=DIRECTION('center_axis',(0.,0.,1.));
#14320=DIRECTION('ref_axis',(1.,0.,0.));
#14321=DIRECTION('center_axis',(0.,-1.,0.));
#14322=DIRECTION('ref_axis',(0.,0.,-1.));
#14323=DIRECTION('center_axis',(0.,1.,0.));
#14324=DIRECTION('ref_axis',(1.,0.,0.));
#14325=DIRECTION('center_axis',(0.,1.,0.));
#14326=DIRECTION('ref_axis',(1.,0.,0.));
#14327=DIRECTION('',(0.,1.,0.));
#14328=DIRECTION('center_axis',(0.,-1.,0.));
#14329=DIRECTION('ref_axis',(1.,0.,0.));
#14330=DIRECTION('center_axis',(0.,-1.,0.));
#14331=DIRECTION('ref_axis',(1.,0.,0.));
#14332=DIRECTION('center_axis',(0.,1.,0.));
#14333=DIRECTION('ref_axis',(1.,0.,0.));
#14334=DIRECTION('center_axis',(0.,-1.,0.));
#14335=DIRECTION('ref_axis',(0.,0.,-1.));
#14336=DIRECTION('center_axis',(0.,0.,1.));
#14337=DIRECTION('ref_axis',(1.,0.,0.));
#14338=DIRECTION('center_axis',(0.,-1.,0.));
#14339=DIRECTION('ref_axis',(0.,0.,-1.));
#14340=DIRECTION('center_axis',(0.,-1.,0.));
#14341=DIRECTION('ref_axis',(-1.,0.,0.));
#14342=DIRECTION('center_axis',(0.,1.,0.));
#14343=DIRECTION('ref_axis',(1.,0.,0.));
#17328=CARTESIAN_POINT('',(0.,0.,0.));
#17329=CARTESIAN_POINT('Origin',(1.18440385848747,0.,1.18440385848747));
#17330=CARTESIAN_POINT('',(0.846804978391753,-0.07938,1.40825612658882));
#17331=CARTESIAN_POINT('',(1.40825612658882,-0.07938,0.846804978391754));
#17332=CARTESIAN_POINT('Ctrl Pts',(0.846804978391752,-0.0793800000000001,
1.40825612658882));
#17333=CARTESIAN_POINT('Ctrl Pts',(0.854205272175554,-0.123401821157026,
1.40380622184538));
#17334=CARTESIAN_POINT('Ctrl Pts',(0.867957148219441,-0.166543350814306,
1.39550172959303));
#17335=CARTESIAN_POINT('Ctrl Pts',(0.902193646979982,-0.237231147975234,
1.3735491215176));
#17336=CARTESIAN_POINT('Ctrl Pts',(0.920778333482564,-0.266264900654909,
1.36127834356734));
#17337=CARTESIAN_POINT('Ctrl Pts',(0.962485392528369,-0.317195968905306,
1.33211611256184));
#17338=CARTESIAN_POINT('Ctrl Pts',(0.985600426557816,-0.33909093068465,
1.31521005565926));
#17339=CARTESIAN_POINT('Ctrl Pts',(1.03253285680459,-0.373586846396559,
1.27866649102984));
#17340=CARTESIAN_POINT('Ctrl Pts',(1.05871835910697,-0.388086240756494,
1.25722555095714));
#17341=CARTESIAN_POINT('Ctrl Pts',(1.11153475808518,-0.407068917407805,
1.2107812086231));
#17342=CARTESIAN_POINT('Ctrl Pts',(1.13814686046673,-0.411552957311693,
1.18575674747573));
#17343=CARTESIAN_POINT('Ctrl Pts',(1.18575674747573,-0.411552957311693,
1.13814686046673));
#17344=CARTESIAN_POINT('Ctrl Pts',(1.2107812086231,-0.407068917407805,1.11153475808518));
#17345=CARTESIAN_POINT('Ctrl Pts',(1.25722555095713,-0.388086240756494,
1.05871835910697));
#17346=CARTESIAN_POINT('Ctrl Pts',(1.27866649102984,-0.373586846396559,
1.03253285680459));
#17347=CARTESIAN_POINT('Ctrl Pts',(1.31521005565926,-0.33909093068465,0.985600426557816));
#17348=CARTESIAN_POINT('Ctrl Pts',(1.33211611256184,-0.317195968905306,
0.962485392528369));
#17349=CARTESIAN_POINT('Ctrl Pts',(1.36127834356734,-0.266264900654909,
0.920778333482565));
#17350=CARTESIAN_POINT('Ctrl Pts',(1.3735491215176,-0.237231147975234,0.902193646979983));
#17351=CARTESIAN_POINT('Ctrl Pts',(1.39550172959303,-0.166543350814306,
0.867957148219442));
#17352=CARTESIAN_POINT('Ctrl Pts',(1.40380622184538,-0.123401821157026,
0.854205272175555));
#17353=CARTESIAN_POINT('Ctrl Pts',(1.40825612658882,-0.0793800000000001,
0.846804978391753));
#17354=CARTESIAN_POINT('',(0.886256117232623,-0.07938,1.45861320581289));
#17355=CARTESIAN_POINT('Origin',(1.18440385848747,-0.07938,1.18440385848747));
#17356=CARTESIAN_POINT('',(1.45861320581289,-0.07938,0.886256117232624));
#17357=CARTESIAN_POINT('Ctrl Pts',(1.45861320581289,-0.0793800000000001,
0.886256117232623));
#17358=CARTESIAN_POINT('Ctrl Pts',(1.45630208793976,-0.101649918886749,
0.890059788636852));
#17359=CARTESIAN_POINT('Ctrl Pts',(1.45296717977858,-0.123823518623746,
0.895520212222107));
#17360=CARTESIAN_POINT('Ctrl Pts',(1.43904931717599,-0.192480977588836,
0.917859913453975));
#17361=CARTESIAN_POINT('Ctrl Pts',(1.4243271592157,-0.236152929235938,0.940896403863072));
#17362=CARTESIAN_POINT('Ctrl Pts',(1.39055359345152,-0.303141259068212,
0.990027513266106));
#17363=CARTESIAN_POINT('Ctrl Pts',(1.36743459453896,-0.335108247315849,
1.02199477007745));
#17364=CARTESIAN_POINT('Ctrl Pts',(1.32643091652006,-0.373243761060364,
1.07446535104584));
#17365=CARTESIAN_POINT('Ctrl Pts',(1.30441816675528,-0.387888272594439,
1.10126842659597));
#17366=CARTESIAN_POINT('Ctrl Pts',(1.25681160160691,-0.407041111792943,
1.15530234155453));
#17367=CARTESIAN_POINT('Ctrl Pts',(1.23119764287622,-0.411552957311693,
1.18251418313119));
#17368=CARTESIAN_POINT('Ctrl Pts',(1.18251418313119,-0.411552957311693,
1.23119764287622));
#17369=CARTESIAN_POINT('Ctrl Pts',(1.15530234155453,-0.407041111792943,
1.25681160160691));
#17370=CARTESIAN_POINT('Ctrl Pts',(1.10126842659597,-0.387888272594439,
1.30441816675528));
#17371=CARTESIAN_POINT('Ctrl Pts',(1.07446535104584,-0.373243761060364,
1.32643091652006));
#17372=CARTESIAN_POINT('Ctrl Pts',(1.02199477007745,-0.335108247315848,
1.36743459453896));
#17373=CARTESIAN_POINT('Ctrl Pts',(0.990027513266105,-0.303141259068211,
1.39055359345152));
#17374=CARTESIAN_POINT('Ctrl Pts',(0.940896403863071,-0.236152929235937,
1.42432715921571));
#17375=CARTESIAN_POINT('Ctrl Pts',(0.917859913453974,-0.192480977588835,
1.43904931717599));
#17376=CARTESIAN_POINT('Ctrl Pts',(0.895520212222106,-0.123823518623745,
1.45296717977858));
#17377=CARTESIAN_POINT('Ctrl Pts',(0.890059788636851,-0.101649918886749,
1.45630208793976));
#17378=CARTESIAN_POINT('Ctrl Pts',(0.886256117232622,-0.0793800000000001,
1.45861320581289));
#17379=CARTESIAN_POINT('Origin',(1.18440385848747,-0.07938,1.18440385848747));
#17380=CARTESIAN_POINT('Origin',(0.,-0.27783,0.));
#17381=CARTESIAN_POINT('',(0.404717578595295,-0.07938,1.65807299932179));
#17382=CARTESIAN_POINT('Origin',(0.,-0.07938,0.));
#17383=CARTESIAN_POINT('',(-0.404717578595296,-0.07938,1.65807299932179));
#17384=CARTESIAN_POINT('Ctrl Pts',(0.404717578595296,-0.0793800000000001,
1.65807299932179));
#17385=CARTESIAN_POINT('Ctrl Pts',(0.400393769631747,-0.101649918886749,
1.65912839404491));
#17386=CARTESIAN_POINT('Ctrl Pts',(0.394174530911058,-0.123823518623745,
1.66063136041479));
#17387=CARTESIAN_POINT('Ctrl Pts',(0.368536561654407,-0.192480977588835,
1.66658649961961));
#17388=CARTESIAN_POINT('Ctrl Pts',(0.341837165343982,-0.236152929235937,
1.67246562047521));
#17389=CARTESIAN_POINT('Ctrl Pts',(0.283214707341173,-0.303141259068211,
1.68332504372461));
#17390=CARTESIAN_POINT('Ctrl Pts',(0.244262842368623,-0.335108247315849,
1.68958170688653));
#17391=CARTESIAN_POINT('Ctrl Pts',(0.178166559972324,-0.373243761060364,
1.69769003172132));
#17392=CARTESIAN_POINT('Ctrl Pts',(0.143648558862931,-0.387888272594439,
1.70107730356824));
#17393=CARTESIAN_POINT('Ctrl Pts',(0.0717778861362652,-0.407041111792943,
1.70562212620408));
#17394=CARTESIAN_POINT('Ctrl Pts',(0.0344244045173309,-0.411552957311693,
1.706752));
#17395=CARTESIAN_POINT('Ctrl Pts',(-0.0344244045173315,-0.411552957311693,
1.706752));
#17396=CARTESIAN_POINT('Ctrl Pts',(-0.0717778861362658,-0.407041111792943,
1.70562212620408));
#17397=CARTESIAN_POINT('Ctrl Pts',(-0.143648558862932,-0.387888272594439,
1.70107730356824));
#17398=CARTESIAN_POINT('Ctrl Pts',(-0.178166559972325,-0.373243761060364,
1.69769003172132));
#17399=CARTESIAN_POINT('Ctrl Pts',(-0.244262842368624,-0.335108247315849,
1.68958170688653));
#17400=CARTESIAN_POINT('Ctrl Pts',(-0.283214707341173,-0.303141259068212,
1.68332504372461));
#17401=CARTESIAN_POINT('Ctrl Pts',(-0.341837165343982,-0.236152929235937,
1.67246562047521));
#17402=CARTESIAN_POINT('Ctrl Pts',(-0.368536561654408,-0.192480977588835,
1.66658649961961));
#17403=CARTESIAN_POINT('Ctrl Pts',(-0.394174530911059,-0.123823518623745,
1.66063136041479));
#17404=CARTESIAN_POINT('Ctrl Pts',(-0.400393769631748,-0.101649918886749,
1.65912839404491));
#17405=CARTESIAN_POINT('Ctrl Pts',(-0.404717578595297,-0.0793800000000001,
1.65807299932179));
#17406=CARTESIAN_POINT('',(-0.886256117232624,-0.07938,1.45861320581289));
#17407=CARTESIAN_POINT('Origin',(0.,-0.07938,0.));
#17408=CARTESIAN_POINT('',(-1.45861320581289,-0.07938,0.886256117232623));
#17409=CARTESIAN_POINT('Ctrl Pts',(-0.886256117232623,-0.0793800000000001,
1.45861320581289));
#17410=CARTESIAN_POINT('Ctrl Pts',(-0.890059788636852,-0.101649918886749,
1.45630208793976));
#17411=CARTESIAN_POINT('Ctrl Pts',(-0.895520212222106,-0.123823518623745,
1.45296717977858));
#17412=CARTESIAN_POINT('Ctrl Pts',(-0.917859913453974,-0.192480977588835,
1.43904931717599));
#17413=CARTESIAN_POINT('Ctrl Pts',(-0.940896403863071,-0.236152929235937,
1.4243271592157));
#17414=CARTESIAN_POINT('Ctrl Pts',(-0.990027513266105,-0.303141259068211,
1.39055359345152));
#17415=CARTESIAN_POINT('Ctrl Pts',(-1.02199477007745,-0.335108247315848,
1.36743459453896));
#17416=CARTESIAN_POINT('Ctrl Pts',(-1.07446535104584,-0.373243761060364,
1.32643091652006));
#17417=CARTESIAN_POINT('Ctrl Pts',(-1.10126842659597,-0.387888272594439,
1.30441816675528));
#17418=CARTESIAN_POINT('Ctrl Pts',(-1.15530234155453,-0.407041111792943,
1.25681160160691));
#17419=CARTESIAN_POINT('Ctrl Pts',(-1.18251418313119,-0.411552957311693,
1.23119764287622));
#17420=CARTESIAN_POINT('Ctrl Pts',(-1.23119764287622,-0.411552957311693,
1.18251418313119));
#17421=CARTESIAN_POINT('Ctrl Pts',(-1.25681160160691,-0.407041111792943,
1.15530234155453));
#17422=CARTESIAN_POINT('Ctrl Pts',(-1.30441816675528,-0.387888272594439,
1.10126842659597));
#17423=CARTESIAN_POINT('Ctrl Pts',(-1.32643091652006,-0.373243761060365,
1.07446535104584));
#17424=CARTESIAN_POINT('Ctrl Pts',(-1.36743459453896,-0.335108247315849,
1.02199477007745));
#17425=CARTESIAN_POINT('Ctrl Pts',(-1.39055359345152,-0.303141259068212,
0.990027513266106));
#17426=CARTESIAN_POINT('Ctrl Pts',(-1.4243271592157,-0.236152929235938,
0.940896403863071));
#17427=CARTESIAN_POINT('Ctrl Pts',(-1.43904931717599,-0.192480977588836,
0.917859913453974));
#17428=CARTESIAN_POINT('Ctrl Pts',(-1.45296717977858,-0.123823518623746,
0.895520212222106));
#17429=CARTESIAN_POINT('Ctrl Pts',(-1.45630208793976,-0.101649918886749,
0.890059788636852));
#17430=CARTESIAN_POINT('Ctrl Pts',(-1.45861320581289,-0.0793800000000001,
0.886256117232623));
#17431=CARTESIAN_POINT('',(-1.65807299932179,-0.07938,0.404717578595295));
#17432=CARTESIAN_POINT('Origin',(0.,-0.07938,0.));
#17433=CARTESIAN_POINT('',(-1.706752,-0.411552957311693,2.08591827245526E-16));
#17434=CARTESIAN_POINT('Ctrl Pts',(-1.65807299932179,-0.0793800000000001,
0.404717578595296));
#17435=CARTESIAN_POINT('Ctrl Pts',(-1.65912839404491,-0.101649918886749,
0.400393769631747));
#17436=CARTESIAN_POINT('Ctrl Pts',(-1.66063136041479,-0.123823518623745,
0.394174530911058));
#17437=CARTESIAN_POINT('Ctrl Pts',(-1.66658649961961,-0.192480977588835,
0.368536561654407));
#17438=CARTESIAN_POINT('Ctrl Pts',(-1.67246562047521,-0.236152929235937,
0.341837165343982));
#17439=CARTESIAN_POINT('Ctrl Pts',(-1.68332504372461,-0.303141259068211,
0.283214707341173));
#17440=CARTESIAN_POINT('Ctrl Pts',(-1.68958170688653,-0.335108247315848,
0.244262842368623));
#17441=CARTESIAN_POINT('Ctrl Pts',(-1.69769003172132,-0.373243761060364,
0.178166559972324));
#17442=CARTESIAN_POINT('Ctrl Pts',(-1.70107730356824,-0.387888272594439,
0.143648558862931));
#17443=CARTESIAN_POINT('Ctrl Pts',(-1.70562212620408,-0.407041111792943,
0.0717778861362656));
#17444=CARTESIAN_POINT('Ctrl Pts',(-1.706752,-0.411552957311693,0.0344244045173313));
#17445=CARTESIAN_POINT('Ctrl Pts',(-1.706752,-0.411552957311693,2.08166817117217E-16));
#17446=CARTESIAN_POINT('',(-1.706752,-0.47628,2.09016837373834E-16));
#17447=CARTESIAN_POINT('',(-1.706752,-0.27783,2.09016837373834E-16));
#17448=CARTESIAN_POINT('Origin',(0.,-0.47628,0.));
#17449=CARTESIAN_POINT('',(-1.65807299932179,-0.07938,-0.404717578595296));
#17450=CARTESIAN_POINT('Ctrl Pts',(-1.706752,-0.411552957311693,2.0122792321331E-16));
#17451=CARTESIAN_POINT('Ctrl Pts',(-1.706752,-0.411552957311693,-0.0344244045173309));
#17452=CARTESIAN_POINT('Ctrl Pts',(-1.70562212620408,-0.407041111792943,
-0.0717778861362652));
#17453=CARTESIAN_POINT('Ctrl Pts',(-1.70107730356824,-0.387888272594439,
-0.143648558862931));
#17454=CARTESIAN_POINT('Ctrl Pts',(-1.69769003172132,-0.373243761060365,
-0.178166559972324));
#17455=CARTESIAN_POINT('Ctrl Pts',(-1.68958170688653,-0.335108247315849,
-0.244262842368623));
#17456=CARTESIAN_POINT('Ctrl Pts',(-1.68332504372461,-0.303141259068212,
-0.283214707341173));
#17457=CARTESIAN_POINT('Ctrl Pts',(-1.67246562047521,-0.236152929235938,
-0.341837165343982));
#17458=CARTESIAN_POINT('Ctrl Pts',(-1.66658649961961,-0.192480977588836,
-0.368536561654407));
#17459=CARTESIAN_POINT('Ctrl Pts',(-1.66063136041479,-0.123823518623745,
-0.394174530911059));
#17460=CARTESIAN_POINT('Ctrl Pts',(-1.65912839404491,-0.101649918886749,
-0.400393769631748));
#17461=CARTESIAN_POINT('Ctrl Pts',(-1.65807299932179,-0.0793800000000001,
-0.404717578595296));
#17462=CARTESIAN_POINT('',(-1.45861320581289,-0.07938,-0.886256117232623));
#17463=CARTESIAN_POINT('Origin',(0.,-0.07938,0.));
#17464=CARTESIAN_POINT('',(-0.886256117232623,-0.07938,-1.45861320581289));
#17465=CARTESIAN_POINT('Ctrl Pts',(-1.45861320581289,-0.0793800000000001,
-0.886256117232623));
#17466=CARTESIAN_POINT('Ctrl Pts',(-1.45630208793976,-0.101649918886749,
-0.890059788636852));
#17467=CARTESIAN_POINT('Ctrl Pts',(-1.45296717977858,-0.123823518623745,
-0.895520212222106));
#17468=CARTESIAN_POINT('Ctrl Pts',(-1.43904931717599,-0.192480977588835,
-0.917859913453974));
#17469=CARTESIAN_POINT('Ctrl Pts',(-1.4243271592157,-0.236152929235937,
-0.940896403863072));
#17470=CARTESIAN_POINT('Ctrl Pts',(-1.39055359345152,-0.303141259068212,
-0.990027513266106));
#17471=CARTESIAN_POINT('Ctrl Pts',(-1.36743459453896,-0.335108247315849,
-1.02199477007745));
#17472=CARTESIAN_POINT('Ctrl Pts',(-1.32643091652006,-0.373243761060364,
-1.07446535104584));
#17473=CARTESIAN_POINT('Ctrl Pts',(-1.30441816675528,-0.387888272594439,
-1.10126842659597));
#17474=CARTESIAN_POINT('Ctrl Pts',(-1.25681160160691,-0.407041111792943,
-1.15530234155453));
#17475=CARTESIAN_POINT('Ctrl Pts',(-1.23119764287622,-0.411552957311693,
-1.18251418313119));
#17476=CARTESIAN_POINT('Ctrl Pts',(-1.18251418313119,-0.411552957311693,
-1.23119764287622));
#17477=CARTESIAN_POINT('Ctrl Pts',(-1.15530234155453,-0.407041111792943,
-1.25681160160691));
#17478=CARTESIAN_POINT('Ctrl Pts',(-1.10126842659597,-0.387888272594439,
-1.30441816675528));
#17479=CARTESIAN_POINT('Ctrl Pts',(-1.07446535104584,-0.373243761060364,
-1.32643091652006));
#17480=CARTESIAN_POINT('Ctrl Pts',(-1.02199477007745,-0.335108247315848,
-1.36743459453896));
#17481=CARTESIAN_POINT('Ctrl Pts',(-0.990027513266105,-0.303141259068211,
-1.39055359345152));
#17482=CARTESIAN_POINT('Ctrl Pts',(-0.940896403863071,-0.236152929235936,
-1.42432715921571));
#17483=CARTESIAN_POINT('Ctrl Pts',(-0.917859913453974,-0.192480977588835,
-1.43904931717599));
#17484=CARTESIAN_POINT('Ctrl Pts',(-0.895520212222106,-0.123823518623745,
-1.45296717977858));
#17485=CARTESIAN_POINT('Ctrl Pts',(-0.890059788636851,-0.101649918886749,
-1.45630208793976));
#17486=CARTESIAN_POINT('Ctrl Pts',(-0.886256117232623,-0.0793800000000001,
-1.45861320581289));
#17487=CARTESIAN_POINT('',(-0.404717578595295,-0.07938,-1.65807299932179));
#17488=CARTESIAN_POINT('Origin',(0.,-0.07938,0.));
#17489=CARTESIAN_POINT('',(0.404717578595296,-0.07938,-1.65807299932179));
#17490=CARTESIAN_POINT('Ctrl Pts',(-0.404717578595296,-0.0793800000000001,
-1.65807299932179));
#17491=CARTESIAN_POINT('Ctrl Pts',(-0.400393769631747,-0.101649918886749,
-1.65912839404491));
#17492=CARTESIAN_POINT('Ctrl Pts',(-0.394174530911058,-0.123823518623746,
-1.66063136041479));
#17493=CARTESIAN_POINT('Ctrl Pts',(-0.368536561654407,-0.192480977588836,
-1.66658649961961));
#17494=CARTESIAN_POINT('Ctrl Pts',(-0.341837165343982,-0.236152929235938,
-1.67246562047521));
#17495=CARTESIAN_POINT('Ctrl Pts',(-0.283214707341173,-0.303141259068212,
-1.68332504372461));
#17496=CARTESIAN_POINT('Ctrl Pts',(-0.244262842368623,-0.335108247315849,
-1.68958170688653));
#17497=CARTESIAN_POINT('Ctrl Pts',(-0.178166559972324,-0.373243761060364,
-1.69769003172132));
#17498=CARTESIAN_POINT('Ctrl Pts',(-0.143648558862931,-0.387888272594439,
-1.70107730356824));
#17499=CARTESIAN_POINT('Ctrl Pts',(-0.0717778861362653,-0.407041111792943,
-1.70562212620408));
#17500=CARTESIAN_POINT('Ctrl Pts',(-0.034424404517331,-0.411552957311693,
-1.706752));
#17501=CARTESIAN_POINT('Ctrl Pts',(0.0344244045173312,-0.411552957311693,
-1.706752));
#17502=CARTESIAN_POINT('Ctrl Pts',(0.0717778861362655,-0.407041111792943,
-1.70562212620408));
#17503=CARTESIAN_POINT('Ctrl Pts',(0.143648558862931,-0.387888272594439,
-1.70107730356824));
#17504=CARTESIAN_POINT('Ctrl Pts',(0.178166559972324,-0.373243761060364,
-1.69769003172132));
#17505=CARTESIAN_POINT('Ctrl Pts',(0.244262842368623,-0.335108247315849,
-1.68958170688653));
#17506=CARTESIAN_POINT('Ctrl Pts',(0.283214707341173,-0.303141259068212,
-1.68332504372461));
#17507=CARTESIAN_POINT('Ctrl Pts',(0.341837165343982,-0.236152929235937,
-1.67246562047521));
#17508=CARTESIAN_POINT('Ctrl Pts',(0.368536561654407,-0.192480977588835,
-1.66658649961961));
#17509=CARTESIAN_POINT('Ctrl Pts',(0.394174530911059,-0.123823518623745,
-1.66063136041479));
#17510=CARTESIAN_POINT('Ctrl Pts',(0.400393769631748,-0.101649918886749,
-1.65912839404491));
#17511=CARTESIAN_POINT('Ctrl Pts',(0.404717578595296,-0.0793800000000001,
-1.65807299932179));
#17512=CARTESIAN_POINT('',(0.886256117232623,-0.07938,-1.45861320581289));
#17513=CARTESIAN_POINT('Origin',(0.,-0.07938,0.));
#17514=CARTESIAN_POINT('',(1.45861320581289,-0.07938,-0.886256117232623));
#17515=CARTESIAN_POINT('Ctrl Pts',(0.886256117232623,-0.0793800000000001,
-1.45861320581289));
#17516=CARTESIAN_POINT('Ctrl Pts',(0.890059788636852,-0.101649918886749,
-1.45630208793976));
#17517=CARTESIAN_POINT('Ctrl Pts',(0.895520212222106,-0.123823518623745,
-1.45296717977858));
#17518=CARTESIAN_POINT('Ctrl Pts',(0.917859913453974,-0.192480977588835,
-1.43904931717599));
#17519=CARTESIAN_POINT('Ctrl Pts',(0.940896403863072,-0.236152929235937,
-1.4243271592157));
#17520=CARTESIAN_POINT('Ctrl Pts',(0.990027513266106,-0.303141259068211,
-1.39055359345152));
#17521=CARTESIAN_POINT('Ctrl Pts',(1.02199477007745,-0.335108247315849,
-1.36743459453896));
#17522=CARTESIAN_POINT('Ctrl Pts',(1.07446535104584,-0.373243761060364,
-1.32643091652006));
#17523=CARTESIAN_POINT('Ctrl Pts',(1.10126842659597,-0.387888272594439,
-1.30441816675528));
#17524=CARTESIAN_POINT('Ctrl Pts',(1.15530234155453,-0.407041111792943,
-1.25681160160691));
#17525=CARTESIAN_POINT('Ctrl Pts',(1.18251418313119,-0.411552957311693,
-1.23119764287622));
#17526=CARTESIAN_POINT('Ctrl Pts',(1.23119764287622,-0.411552957311693,
-1.18251418313119));
#17527=CARTESIAN_POINT('Ctrl Pts',(1.25681160160691,-0.407041111792943,
-1.15530234155453));
#17528=CARTESIAN_POINT('Ctrl Pts',(1.30441816675528,-0.387888272594439,
-1.10126842659597));
#17529=CARTESIAN_POINT('Ctrl Pts',(1.32643091652006,-0.373243761060364,
-1.07446535104584));
#17530=CARTESIAN_POINT('Ctrl Pts',(1.36743459453896,-0.335108247315849,
-1.02199477007745));
#17531=CARTESIAN_POINT('Ctrl Pts',(1.39055359345152,-0.303141259068212,
-0.990027513266105));
#17532=CARTESIAN_POINT('Ctrl Pts',(1.4243271592157,-0.236152929235937,-0.940896403863071));
#17533=CARTESIAN_POINT('Ctrl Pts',(1.43904931717599,-0.192480977588835,
-0.917859913453974));
#17534=CARTESIAN_POINT('Ctrl Pts',(1.45296717977858,-0.123823518623745,
-0.895520212222106));
#17535=CARTESIAN_POINT('Ctrl Pts',(1.45630208793976,-0.101649918886749,
-0.890059788636852));
#17536=CARTESIAN_POINT('Ctrl Pts',(1.45861320581289,-0.0793800000000001,
-0.886256117232623));
#17537=CARTESIAN_POINT('',(1.65807299932179,-0.07938,-0.404717578595296));
#17538=CARTESIAN_POINT('Origin',(0.,-0.07938,0.));
#17539=CARTESIAN_POINT('',(1.65807299932179,-0.07938,0.404717578595296));
#17540=CARTESIAN_POINT('Ctrl Pts',(1.65807299932179,-0.0793800000000001,
-0.404717578595296));
#17541=CARTESIAN_POINT('Ctrl Pts',(1.65912839404491,-0.101649918886749,
-0.400393769631747));
#17542=CARTESIAN_POINT('Ctrl Pts',(1.66063136041479,-0.123823518623745,
-0.394174530911058));
#17543=CARTESIAN_POINT('Ctrl Pts',(1.66658649961961,-0.192480977588835,
-0.368536561654407));
#17544=CARTESIAN_POINT('Ctrl Pts',(1.67246562047521,-0.236152929235937,
-0.341837165343982));
#17545=CARTESIAN_POINT('Ctrl Pts',(1.68332504372461,-0.303141259068212,
-0.283214707341173));
#17546=CARTESIAN_POINT('Ctrl Pts',(1.68958170688653,-0.335108247315849,
-0.244262842368623));
#17547=CARTESIAN_POINT('Ctrl Pts',(1.69769003172132,-0.373243761060364,
-0.178166559972324));
#17548=CARTESIAN_POINT('Ctrl Pts',(1.70107730356824,-0.387888272594439,
-0.143648558862931));
#17549=CARTESIAN_POINT('Ctrl Pts',(1.70562212620408,-0.407041111792943,
-0.0717778861362655));
#17550=CARTESIAN_POINT('Ctrl Pts',(1.706752,-0.411552957311693,-0.0344244045173312));
#17551=CARTESIAN_POINT('Ctrl Pts',(1.706752,-0.411552957311693,0.0344244045173312));
#17552=CARTESIAN_POINT('Ctrl Pts',(1.70562212620408,-0.407041111792943,
0.0717778861362655));
#17553=CARTESIAN_POINT('Ctrl Pts',(1.70107730356824,-0.387888272594439,
0.143648558862931));
#17554=CARTESIAN_POINT('Ctrl Pts',(1.69769003172132,-0.373243761060364,
0.178166559972324));
#17555=CARTESIAN_POINT('Ctrl Pts',(1.68958170688653,-0.335108247315849,
0.244262842368623));
#17556=CARTESIAN_POINT('Ctrl Pts',(1.68332504372461,-0.303141259068212,
0.283214707341173));
#17557=CARTESIAN_POINT('Ctrl Pts',(1.67246562047521,-0.236152929235937,
0.341837165343982));
#17558=CARTESIAN_POINT('Ctrl Pts',(1.66658649961961,-0.192480977588835,
0.368536561654407));
#17559=CARTESIAN_POINT('Ctrl Pts',(1.66063136041479,-0.123823518623745,
0.394174530911058));
#17560=CARTESIAN_POINT('Ctrl Pts',(1.65912839404491,-0.101649918886749,
0.400393769631747));
#17561=CARTESIAN_POINT('Ctrl Pts',(1.65807299932179,-0.0793800000000001,
0.404717578595296));
#17562=CARTESIAN_POINT('Origin',(0.,-0.07938,0.));
#17563=CARTESIAN_POINT('Origin',(0.,-0.07938,0.));
#17564=CARTESIAN_POINT('',(0.397005914195118,-0.07938,1.59456899932179));
#17565=CARTESIAN_POINT('Origin',(0.,-0.07938,0.));
#17566=CARTESIAN_POINT('Origin',(-3.33066907387547E-16,-0.07938,1.675));
#17567=CARTESIAN_POINT('Origin',(-3.33066907387547E-16,0.,1.675));
#17568=CARTESIAN_POINT('',(-0.397005914195118,-0.07938,1.59456899932179));
#17569=CARTESIAN_POINT('Ctrl Pts',(-0.397005914195119,-0.0793800000000001,
1.59456899932179));
#17570=CARTESIAN_POINT('Ctrl Pts',(-0.3886265584581,-0.123401821157026,
1.59665523941937));
#17571=CARTESIAN_POINT('Ctrl Pts',(-0.373030350867485,-0.166543350814306,
1.60050712143809));
#17572=CARTESIAN_POINT('Ctrl Pts',(-0.333298652394954,-0.237231147975234,
1.60919314384089));
#17573=CARTESIAN_POINT('Ctrl Pts',(-0.311480544243687,-0.266264900654909,
1.61365775139403));
#17574=CARTESIAN_POINT('Ctrl Pts',(-0.261368388670537,-0.317195968905306,
1.62252828437015));
#17575=CARTESIAN_POINT('Ctrl Pts',(-0.233069203882014,-0.33909093068465,
1.62691869420078));
#17576=CARTESIAN_POINT('Ctrl Pts',(-0.174042761838764,-0.373586846396559,
1.63426473152765));
#17577=CARTESIAN_POINT('Ctrl Pts',(-0.14036578147155,-0.388086240756494,
1.63761964365402));
#17578=CARTESIAN_POINT('Ctrl Pts',(-0.0701778381840615,-0.407068917407805,
1.64212536811722));
#17579=CARTESIAN_POINT('Ctrl Pts',(-0.0336652739555918,-0.411552957311693,
1.643248));
#17580=CARTESIAN_POINT('Ctrl Pts',(0.0336652739555913,-0.411552957311693,
1.643248));
#17581=CARTESIAN_POINT('Ctrl Pts',(0.070177838184061,-0.407068917407805,
1.64212536811722));
#17582=CARTESIAN_POINT('Ctrl Pts',(0.140365781471549,-0.388086240756494,
1.63761964365402));
#17583=CARTESIAN_POINT('Ctrl Pts',(0.174042761838763,-0.373586846396559,
1.63426473152765));
#17584=CARTESIAN_POINT('Ctrl Pts',(0.233069203882014,-0.33909093068465,
1.62691869420078));
#17585=CARTESIAN_POINT('Ctrl Pts',(0.261368388670536,-0.317195968905306,
1.62252828437015));
#17586=CARTESIAN_POINT('Ctrl Pts',(0.311480544243686,-0.266264900654908,
1.61365775139403));
#17587=CARTESIAN_POINT('Ctrl Pts',(0.333298652394954,-0.237231147975234,
1.60919314384089));
#17588=CARTESIAN_POINT('Ctrl Pts',(0.373030350867484,-0.166543350814306,
1.60050712143809));
#17589=CARTESIAN_POINT('Ctrl Pts',(0.388626558458099,-0.123401821157026,
1.59665523941937));
#17590=CARTESIAN_POINT('Ctrl Pts',(0.397005914195118,-0.07938,1.59456899932179));
#17591=CARTESIAN_POINT('Origin',(-3.33066907387547E-16,-0.07938,1.675));
#17592=CARTESIAN_POINT('Origin',(0.,-0.07938,0.));
#17593=CARTESIAN_POINT('',(-0.846804978391754,-0.07938,1.40825612658882));
#17594=CARTESIAN_POINT('Origin',(0.,-0.07938,0.));
#17595=CARTESIAN_POINT('Origin',(-1.18440385848747,-0.07938,1.18440385848747));
#17596=CARTESIAN_POINT('Origin',(-1.18440385848747,0.,1.18440385848747));
#17597=CARTESIAN_POINT('',(-1.40825612658882,-0.07938,0.846804978391753));
#17598=CARTESIAN_POINT('Ctrl Pts',(-1.40825612658882,-0.0793800000000001,
0.846804978391753));
#17599=CARTESIAN_POINT('Ctrl Pts',(-1.40380622184538,-0.123401821157026,
0.854205272175555));
#17600=CARTESIAN_POINT('Ctrl Pts',(-1.39550172959303,-0.166543350814306,
0.867957148219442));
#17601=CARTESIAN_POINT('Ctrl Pts',(-1.3735491215176,-0.237231147975235,
0.902193646979983));
#17602=CARTESIAN_POINT('Ctrl Pts',(-1.36127834356734,-0.266264900654909,
0.920778333482565));
#17603=CARTESIAN_POINT('Ctrl Pts',(-1.33211611256184,-0.317195968905306,
0.962485392528369));
#17604=CARTESIAN_POINT('Ctrl Pts',(-1.31521005565926,-0.339090930684651,
0.985600426557816));
#17605=CARTESIAN_POINT('Ctrl Pts',(-1.27866649102984,-0.373586846396559,
1.03253285680459));
#17606=CARTESIAN_POINT('Ctrl Pts',(-1.25722555095714,-0.388086240756494,
1.05871835910697));
#17607=CARTESIAN_POINT('Ctrl Pts',(-1.2107812086231,-0.407068917407805,
1.11153475808518));
#17608=CARTESIAN_POINT('Ctrl Pts',(-1.18575674747573,-0.411552957311693,
1.13814686046673));
#17609=CARTESIAN_POINT('Ctrl Pts',(-1.13814686046673,-0.411552957311693,
1.18575674747573));
#17610=CARTESIAN_POINT('Ctrl Pts',(-1.11153475808518,-0.407068917407805,
1.2107812086231));
#17611=CARTESIAN_POINT('Ctrl Pts',(-1.05871835910697,-0.388086240756494,
1.25722555095714));
#17612=CARTESIAN_POINT('Ctrl Pts',(-1.03253285680459,-0.373586846396559,
1.27866649102984));
#17613=CARTESIAN_POINT('Ctrl Pts',(-0.985600426557816,-0.33909093068465,
1.31521005565926));
#17614=CARTESIAN_POINT('Ctrl Pts',(-0.962485392528369,-0.317195968905306,
1.33211611256184));
#17615=CARTESIAN_POINT('Ctrl Pts',(-0.920778333482565,-0.266264900654908,
1.36127834356734));
#17616=CARTESIAN_POINT('Ctrl Pts',(-0.902193646979983,-0.237231147975234,
1.3735491215176));
#17617=CARTESIAN_POINT('Ctrl Pts',(-0.867957148219442,-0.166543350814306,
1.39550172959303));
#17618=CARTESIAN_POINT('Ctrl Pts',(-0.854205272175555,-0.123401821157026,
1.40380622184538));
#17619=CARTESIAN_POINT('Ctrl Pts',(-0.846804978391753,-0.0793800000000001,
1.40825612658882));
#17620=CARTESIAN_POINT('Origin',(-1.18440385848747,-0.07938,1.18440385848747));
#17621=CARTESIAN_POINT('Origin',(0.,-0.07938,0.));
#17622=CARTESIAN_POINT('',(-1.59456899932179,-0.07938,0.397005914195118));
#17623=CARTESIAN_POINT('Origin',(0.,-0.07938,0.));
#17624=CARTESIAN_POINT('Origin',(-1.675,-0.07938,-2.22044604925031E-16));
#17625=CARTESIAN_POINT('Origin',(-1.675,0.,-2.22044604925031E-16));
#17626=CARTESIAN_POINT('',(-1.59456899932179,-0.07938,-0.397005914195118));
#17627=CARTESIAN_POINT('',(-1.643248,-0.411552957311693,3.47540551556327E-18));
#17628=CARTESIAN_POINT('Ctrl Pts',(-1.59456899932179,-0.0793800000000001,
-0.397005914195119));
#17629=CARTESIAN_POINT('Ctrl Pts',(-1.59665523941937,-0.123401821157026,
-0.388626558458099));
#17630=CARTESIAN_POINT('Ctrl Pts',(-1.60050712143809,-0.166543350814306,
-0.373030350867485));
#17631=CARTESIAN_POINT('Ctrl Pts',(-1.60919314384089,-0.237231147975234,
-0.333298652394954));
#17632=CARTESIAN_POINT('Ctrl Pts',(-1.61365775139403,-0.266264900654909,
-0.311480544243686));
#17633=CARTESIAN_POINT('Ctrl Pts',(-1.62252828437015,-0.317195968905306,
-0.261368388670537));
#17634=CARTESIAN_POINT('Ctrl Pts',(-1.62691869420078,-0.33909093068465,
-0.233069203882014));
#17635=CARTESIAN_POINT('Ctrl Pts',(-1.63426473152765,-0.373586846396559,
-0.174042761838764));
#17636=CARTESIAN_POINT('Ctrl Pts',(-1.63761964365402,-0.388086240756494,
-0.140365781471549));
#17637=CARTESIAN_POINT('Ctrl Pts',(-1.64212536811722,-0.407068917407805,
-0.0701778381840614));
#17638=CARTESIAN_POINT('Ctrl Pts',(-1.643248,-0.411552957311693,-0.0336652739555917));
#17639=CARTESIAN_POINT('Ctrl Pts',(-1.643248,-0.411552957311693,-2.0122792321331E-16));
#17640=CARTESIAN_POINT('Origin',(-1.675,-0.07938,-2.22044604925031E-16));
#17641=CARTESIAN_POINT('Ctrl Pts',(-1.643248,-0.411552957311693,-1.94289029309402E-16));
#17642=CARTESIAN_POINT('Ctrl Pts',(-1.643248,-0.411552957311693,0.0336652739555913));
#17643=CARTESIAN_POINT('Ctrl Pts',(-1.64212536811722,-0.407068917407805,
0.0701778381840609));
#17644=CARTESIAN_POINT('Ctrl Pts',(-1.63761964365402,-0.388086240756494,
0.140365781471549));
#17645=CARTESIAN_POINT('Ctrl Pts',(-1.63426473152765,-0.373586846396559,
0.174042761838763));
#17646=CARTESIAN_POINT('Ctrl Pts',(-1.62691869420078,-0.33909093068465,
0.233069203882014));
#17647=CARTESIAN_POINT('Ctrl Pts',(-1.62252828437015,-0.317195968905306,
0.261368388670536));
#17648=CARTESIAN_POINT('Ctrl Pts',(-1.61365775139403,-0.266264900654909,
0.311480544243686));
#17649=CARTESIAN_POINT('Ctrl Pts',(-1.60919314384089,-0.237231147975235,
0.333298652394954));
#17650=CARTESIAN_POINT('Ctrl Pts',(-1.60050712143809,-0.166543350814306,
0.373030350867484));
#17651=CARTESIAN_POINT('Ctrl Pts',(-1.59665523941937,-0.123401821157026,
0.388626558458099));
#17652=CARTESIAN_POINT('Ctrl Pts',(-1.59456899932179,-0.0793800000000001,
0.397005914195118));
#17653=CARTESIAN_POINT('Origin',(0.,-0.07938,0.));
#17654=CARTESIAN_POINT('',(-1.40825612658882,-0.07938,-0.846804978391753));
#17655=CARTESIAN_POINT('Origin',(0.,-0.07938,0.));
#17656=CARTESIAN_POINT('Origin',(-1.18440385848747,-0.07938,-1.18440385848747));
#17657=CARTESIAN_POINT('Origin',(-1.18440385848747,0.,-1.18440385848747));
#17658=CARTESIAN_POINT('',(-0.846804978391753,-0.07938,-1.40825612658882));
#17659=CARTESIAN_POINT('Ctrl Pts',(-0.846804978391753,-0.0793800000000001,
-1.40825612658882));
#17660=CARTESIAN_POINT('Ctrl Pts',(-0.854205272175555,-0.123401821157026,
-1.40380622184538));
#17661=CARTESIAN_POINT('Ctrl Pts',(-0.867957148219442,-0.166543350814306,
-1.39550172959303));
#17662=CARTESIAN_POINT('Ctrl Pts',(-0.902193646979982,-0.237231147975234,
-1.3735491215176));
#17663=CARTESIAN_POINT('Ctrl Pts',(-0.920778333482564,-0.266264900654908,
-1.36127834356734));
#17664=CARTESIAN_POINT('Ctrl Pts',(-0.962485392528368,-0.317195968905306,
-1.33211611256184));
#17665=CARTESIAN_POINT('Ctrl Pts',(-0.985600426557816,-0.33909093068465,
-1.31521005565926));
#17666=CARTESIAN_POINT('Ctrl Pts',(-1.03253285680459,-0.373586846396559,
-1.27866649102984));
#17667=CARTESIAN_POINT('Ctrl Pts',(-1.05871835910697,-0.388086240756494,
-1.25722555095714));
#17668=CARTESIAN_POINT('Ctrl Pts',(-1.11153475808518,-0.407068917407805,
-1.2107812086231));
#17669=CARTESIAN_POINT('Ctrl Pts',(-1.13814686046673,-0.411552957311693,
-1.18575674747573));
#17670=CARTESIAN_POINT('Ctrl Pts',(-1.18575674747573,-0.411552957311693,
-1.13814686046673));
#17671=CARTESIAN_POINT('Ctrl Pts',(-1.2107812086231,-0.407068917407805,
-1.11153475808518));
#17672=CARTESIAN_POINT('Ctrl Pts',(-1.25722555095714,-0.388086240756494,
-1.05871835910697));
#17673=CARTESIAN_POINT('Ctrl Pts',(-1.27866649102984,-0.373586846396559,
-1.03253285680459));
#17674=CARTESIAN_POINT('Ctrl Pts',(-1.31521005565926,-0.33909093068465,
-0.985600426557816));
#17675=CARTESIAN_POINT('Ctrl Pts',(-1.33211611256184,-0.317195968905306,
-0.962485392528369));
#17676=CARTESIAN_POINT('Ctrl Pts',(-1.36127834356734,-0.266264900654909,
-0.920778333482565));
#17677=CARTESIAN_POINT('Ctrl Pts',(-1.3735491215176,-0.237231147975234,
-0.902193646979983));
#17678=CARTESIAN_POINT('Ctrl Pts',(-1.39550172959303,-0.166543350814306,
-0.867957148219442));
#17679=CARTESIAN_POINT('Ctrl Pts',(-1.40380622184538,-0.123401821157026,
-0.854205272175555));
#17680=CARTESIAN_POINT('Ctrl Pts',(-1.40825612658882,-0.07938,-0.846804978391753));
#17681=CARTESIAN_POINT('Origin',(-1.18440385848747,-0.07938,-1.18440385848747));
#17682=CARTESIAN_POINT('Origin',(0.,-0.07938,0.));
#17683=CARTESIAN_POINT('',(-0.397005914195118,-0.07938,-1.59456899932179));
#17684=CARTESIAN_POINT('Origin',(0.,-0.07938,0.));
#17685=CARTESIAN_POINT('Origin',(1.11022302462516E-16,-0.07938,-1.675));
#17686=CARTESIAN_POINT('Origin',(1.11022302462516E-16,0.,-1.675));
#17687=CARTESIAN_POINT('',(0.397005914195118,-0.07938,-1.59456899932179));
#17688=CARTESIAN_POINT('Ctrl Pts',(0.397005914195119,-0.0793800000000001,
-1.59456899932179));
#17689=CARTESIAN_POINT('Ctrl Pts',(0.388626558458099,-0.123401821157026,
-1.59665523941937));
#17690=CARTESIAN_POINT('Ctrl Pts',(0.373030350867485,-0.166543350814306,
-1.60050712143809));
#17691=CARTESIAN_POINT('Ctrl Pts',(0.333298652394954,-0.237231147975234,
-1.60919314384089));
#17692=CARTESIAN_POINT('Ctrl Pts',(0.311480544243686,-0.266264900654909,
-1.61365775139403));
#17693=CARTESIAN_POINT('Ctrl Pts',(0.261368388670537,-0.317195968905306,
-1.62252828437015));
#17694=CARTESIAN_POINT('Ctrl Pts',(0.233069203882014,-0.33909093068465,
-1.62691869420078));
#17695=CARTESIAN_POINT('Ctrl Pts',(0.174042761838763,-0.373586846396559,
-1.63426473152765));
#17696=CARTESIAN_POINT('Ctrl Pts',(0.140365781471549,-0.388086240756494,
-1.63761964365402));
#17697=CARTESIAN_POINT('Ctrl Pts',(0.0701778381840612,-0.407068917407805,
-1.64212536811722));
#17698=CARTESIAN_POINT('Ctrl Pts',(0.0336652739555916,-0.411552957311693,
-1.643248));
#17699=CARTESIAN_POINT('Ctrl Pts',(-0.0336652739555915,-0.411552957311693,
-1.643248));
#17700=CARTESIAN_POINT('Ctrl Pts',(-0.0701778381840612,-0.407068917407805,
-1.64212536811722));
#17701=CARTESIAN_POINT('Ctrl Pts',(-0.140365781471549,-0.388086240756494,
-1.63761964365402));
#17702=CARTESIAN_POINT('Ctrl Pts',(-0.174042761838764,-0.373586846396559,
-1.63426473152765));
#17703=CARTESIAN_POINT('Ctrl Pts',(-0.233069203882014,-0.33909093068465,
-1.62691869420078));
#17704=CARTESIAN_POINT('Ctrl Pts',(-0.261368388670536,-0.317195968905306,
-1.62252828437015));
#17705=CARTESIAN_POINT('Ctrl Pts',(-0.311480544243686,-0.266264900654908,
-1.61365775139403));
#17706=CARTESIAN_POINT('Ctrl Pts',(-0.333298652394954,-0.237231147975234,
-1.60919314384089));
#17707=CARTESIAN_POINT('Ctrl Pts',(-0.373030350867485,-0.166543350814306,
-1.60050712143809));
#17708=CARTESIAN_POINT('Ctrl Pts',(-0.388626558458099,-0.123401821157026,
-1.59665523941937));
#17709=CARTESIAN_POINT('Ctrl Pts',(-0.397005914195118,-0.07938,-1.59456899932179));
#17710=CARTESIAN_POINT('Origin',(1.11022302462516E-16,-0.07938,-1.675));
#17711=CARTESIAN_POINT('Origin',(0.,-0.07938,0.));
#17712=CARTESIAN_POINT('',(0.846804978391753,-0.07938,-1.40825612658882));
#17713=CARTESIAN_POINT('Origin',(0.,-0.07938,0.));
#17714=CARTESIAN_POINT('Origin',(1.18440385848747,-0.07938,-1.18440385848747));
#17715=CARTESIAN_POINT('Origin',(1.18440385848747,0.,-1.18440385848747));
#17716=CARTESIAN_POINT('',(1.40825612658882,-0.07938,-0.846804978391753));
#17717=CARTESIAN_POINT('Ctrl Pts',(1.40825612658882,-0.0793800000000001,
-0.846804978391753));
#17718=CARTESIAN_POINT('Ctrl Pts',(1.40380622184538,-0.123401821157026,
-0.854205272175555));
#17719=CARTESIAN_POINT('Ctrl Pts',(1.39550172959303,-0.166543350814306,
-0.867957148219442));
#17720=CARTESIAN_POINT('Ctrl Pts',(1.3735491215176,-0.237231147975234,-0.902193646979983));
#17721=CARTESIAN_POINT('Ctrl Pts',(1.36127834356734,-0.266264900654908,
-0.920778333482565));
#17722=CARTESIAN_POINT('Ctrl Pts',(1.33211611256184,-0.317195968905306,
-0.962485392528369));
#17723=CARTESIAN_POINT('Ctrl Pts',(1.31521005565926,-0.33909093068465,-0.985600426557816));
#17724=CARTESIAN_POINT('Ctrl Pts',(1.27866649102984,-0.373586846396559,
-1.03253285680459));
#17725=CARTESIAN_POINT('Ctrl Pts',(1.25722555095714,-0.388086240756494,
-1.05871835910697));
#17726=CARTESIAN_POINT('Ctrl Pts',(1.2107812086231,-0.407068917407805,-1.11153475808518));
#17727=CARTESIAN_POINT('Ctrl Pts',(1.18575674747573,-0.411552957311693,
-1.13814686046673));
#17728=CARTESIAN_POINT('Ctrl Pts',(1.13814686046673,-0.411552957311693,
-1.18575674747573));
#17729=CARTESIAN_POINT('Ctrl Pts',(1.11153475808518,-0.407068917407805,
-1.2107812086231));
#17730=CARTESIAN_POINT('Ctrl Pts',(1.05871835910697,-0.388086240756494,
-1.25722555095714));
#17731=CARTESIAN_POINT('Ctrl Pts',(1.03253285680459,-0.373586846396559,
-1.27866649102984));
#17732=CARTESIAN_POINT('Ctrl Pts',(0.985600426557816,-0.33909093068465,
-1.31521005565926));
#17733=CARTESIAN_POINT('Ctrl Pts',(0.962485392528369,-0.317195968905306,
-1.33211611256184));
#17734=CARTESIAN_POINT('Ctrl Pts',(0.920778333482565,-0.266264900654909,
-1.36127834356734));
#17735=CARTESIAN_POINT('Ctrl Pts',(0.902193646979983,-0.237231147975234,
-1.3735491215176));
#17736=CARTESIAN_POINT('Ctrl Pts',(0.867957148219442,-0.166543350814306,
-1.39550172959303));
#17737=CARTESIAN_POINT('Ctrl Pts',(0.854205272175555,-0.123401821157026,
-1.40380622184538));
#17738=CARTESIAN_POINT('Ctrl Pts',(0.846804978391753,-0.0793800000000001,
-1.40825612658882));
#17739=CARTESIAN_POINT('Origin',(1.18440385848747,-0.07938,-1.18440385848747));
#17740=CARTESIAN_POINT('Origin',(0.,-0.27783,0.));
#17741=CARTESIAN_POINT('',(-1.643248,-0.47628,2.01239840340529E-16));
#17742=CARTESIAN_POINT('Origin',(0.,-0.47628,0.));
#17743=CARTESIAN_POINT('',(-1.643248,-0.27783,2.01239840340529E-16));
#17744=CARTESIAN_POINT('',(1.59456899932179,-0.07938,0.397005914195118));
#17745=CARTESIAN_POINT('Origin',(0.,-0.07938,0.));
#17746=CARTESIAN_POINT('',(1.59456899932179,-0.07938,-0.397005914195118));
#17747=CARTESIAN_POINT('Ctrl Pts',(1.59456899932179,-0.0793800000000001,
0.397005914195118));
#17748=CARTESIAN_POINT('Ctrl Pts',(1.59665523941937,-0.123401821157026,
0.388626558458099));
#17749=CARTESIAN_POINT('Ctrl Pts',(1.60050712143809,-0.166543350814306,
0.373030350867485));
#17750=CARTESIAN_POINT('Ctrl Pts',(1.60919314384089,-0.237231147975234,
0.333298652394954));
#17751=CARTESIAN_POINT('Ctrl Pts',(1.61365775139403,-0.266264900654909,
0.311480544243686));
#17752=CARTESIAN_POINT('Ctrl Pts',(1.62252828437015,-0.317195968905306,
0.261368388670537));
#17753=CARTESIAN_POINT('Ctrl Pts',(1.62691869420078,-0.33909093068465,0.233069203882014));
#17754=CARTESIAN_POINT('Ctrl Pts',(1.63426473152765,-0.373586846396559,
0.174042761838764));
#17755=CARTESIAN_POINT('Ctrl Pts',(1.63761964365402,-0.388086240756494,
0.140365781471549));
#17756=CARTESIAN_POINT('Ctrl Pts',(1.64212536811722,-0.407068917407805,
0.0701778381840612));
#17757=CARTESIAN_POINT('Ctrl Pts',(1.643248,-0.411552957311693,0.0336652739555916));
#17758=CARTESIAN_POINT('Ctrl Pts',(1.643248,-0.411552957311693,-0.0336652739555916));
#17759=CARTESIAN_POINT('Ctrl Pts',(1.64212536811722,-0.407068917407805,
-0.0701778381840612));
#17760=CARTESIAN_POINT('Ctrl Pts',(1.63761964365402,-0.388086240756494,
-0.140365781471549));
#17761=CARTESIAN_POINT('Ctrl Pts',(1.63426473152765,-0.373586846396559,
-0.174042761838764));
#17762=CARTESIAN_POINT('Ctrl Pts',(1.62691869420078,-0.33909093068465,-0.233069203882014));
#17763=CARTESIAN_POINT('Ctrl Pts',(1.62252828437015,-0.317195968905306,
-0.261368388670537));
#17764=CARTESIAN_POINT('Ctrl Pts',(1.61365775139403,-0.266264900654909,
-0.311480544243686));
#17765=CARTESIAN_POINT('Ctrl Pts',(1.60919314384089,-0.237231147975234,
-0.333298652394954));
#17766=CARTESIAN_POINT('Ctrl Pts',(1.60050712143809,-0.166543350814306,
-0.373030350867485));
#17767=CARTESIAN_POINT('Ctrl Pts',(1.59665523941937,-0.123401821157026,
-0.388626558458099));
#17768=CARTESIAN_POINT('Ctrl Pts',(1.59456899932179,-0.07938,-0.397005914195118));
#17769=CARTESIAN_POINT('Origin',(0.,-0.07938,0.));
#17770=CARTESIAN_POINT('Origin',(0.,-0.07938,0.));
#17771=CARTESIAN_POINT('Origin',(1.675,-0.07938,0.));
#17772=CARTESIAN_POINT('Origin',(1.675,0.,0.));
#17773=CARTESIAN_POINT('Origin',(1.675,-0.07938,0.));
#17774=CARTESIAN_POINT('Origin',(0.,-0.47628,0.));
#17775=CARTESIAN_POINT('Origin',(0.,-0.07938,0.));
#53835=UNCERTAINTY_MEASURE_WITH_UNIT(LENGTH_MEASURE(0.001),#53910,
'DISTANCE_ACCURACY_VALUE',
'Maximum model space distance between geometric entities at asserted c
onnectivities');
#53859=UNCERTAINTY_MEASURE_WITH_UNIT(LENGTH_MEASURE(0.001),#53910,
'DISTANCE_ACCURACY_VALUE',
'Maximum model space distance between geometric entities at asserted c
onnectivities');
#53885=(
GEOMETRIC_REPRESENTATION_CONTEXT(3)
GLOBAL_UNCERTAINTY_ASSIGNED_CONTEXT((#53835))
GLOBAL_UNIT_ASSIGNED_CONTEXT((#53910,#53912,#53913))
REPRESENTATION_CONTEXT('','3D')
);
#53909=(
GEOMETRIC_REPRESENTATION_CONTEXT(3)
GLOBAL_UNCERTAINTY_ASSIGNED_CONTEXT((#53859))
GLOBAL_UNIT_ASSIGNED_CONTEXT((#53910,#53912,#53913))
REPRESENTATION_CONTEXT('','3D')
);
#53910=(
LENGTH_UNIT()
NAMED_UNIT(*)
SI_UNIT(.CENTI.,.METRE.)
);
#53912=(
NAMED_UNIT(*)
PLANE_ANGLE_UNIT()
SI_UNIT($,.RADIAN.)
);
#53913=(
NAMED_UNIT(*)
SI_UNIT($,.STERADIAN.)
SOLID_ANGLE_UNIT()
);
#53939=SHAPE_DEFINITION_REPRESENTATION(#53993,#54111);
#53993=PRODUCT_DEFINITION_SHAPE('',$,#54161);
#54111=SHAPE_REPRESENTATION('',(#12339),#53885);
#54135=PRODUCT_DEFINITION_CONTEXT('part definition',#54284,'design');
#54161=PRODUCT_DEFINITION('Cage (1)','Cage (1)',#54210,#54135);
#54210=PRODUCT_DEFINITION_FORMATION('',$,#54311);
#54284=APPLICATION_CONTEXT(
'Core Data for Automotive Mechanical Design Process');
#54285=PRODUCT_CONTEXT('part definition',#54284,'mechanical');
#54311=PRODUCT('Cage (1)','Cage (1)','Cage (1)',(#54285));
#54391=COLOUR_RGB('Grey',0.48,0.52,0.57);
#54392=FILL_AREA_STYLE_COLOUR('',#54391);
#54393=FILL_AREA_STYLE('',(#54392));
#54394=SURFACE_STYLE_FILL_AREA(#54393);
#54395=SURFACE_SIDE_STYLE('',(#54394));
#54396=SURFACE_STYLE_USAGE(.BOTH.,#54395);
#54397=PRESENTATION_STYLE_ASSIGNMENT((#54396));
ENDSEC;
END-ISO-10303-21;
